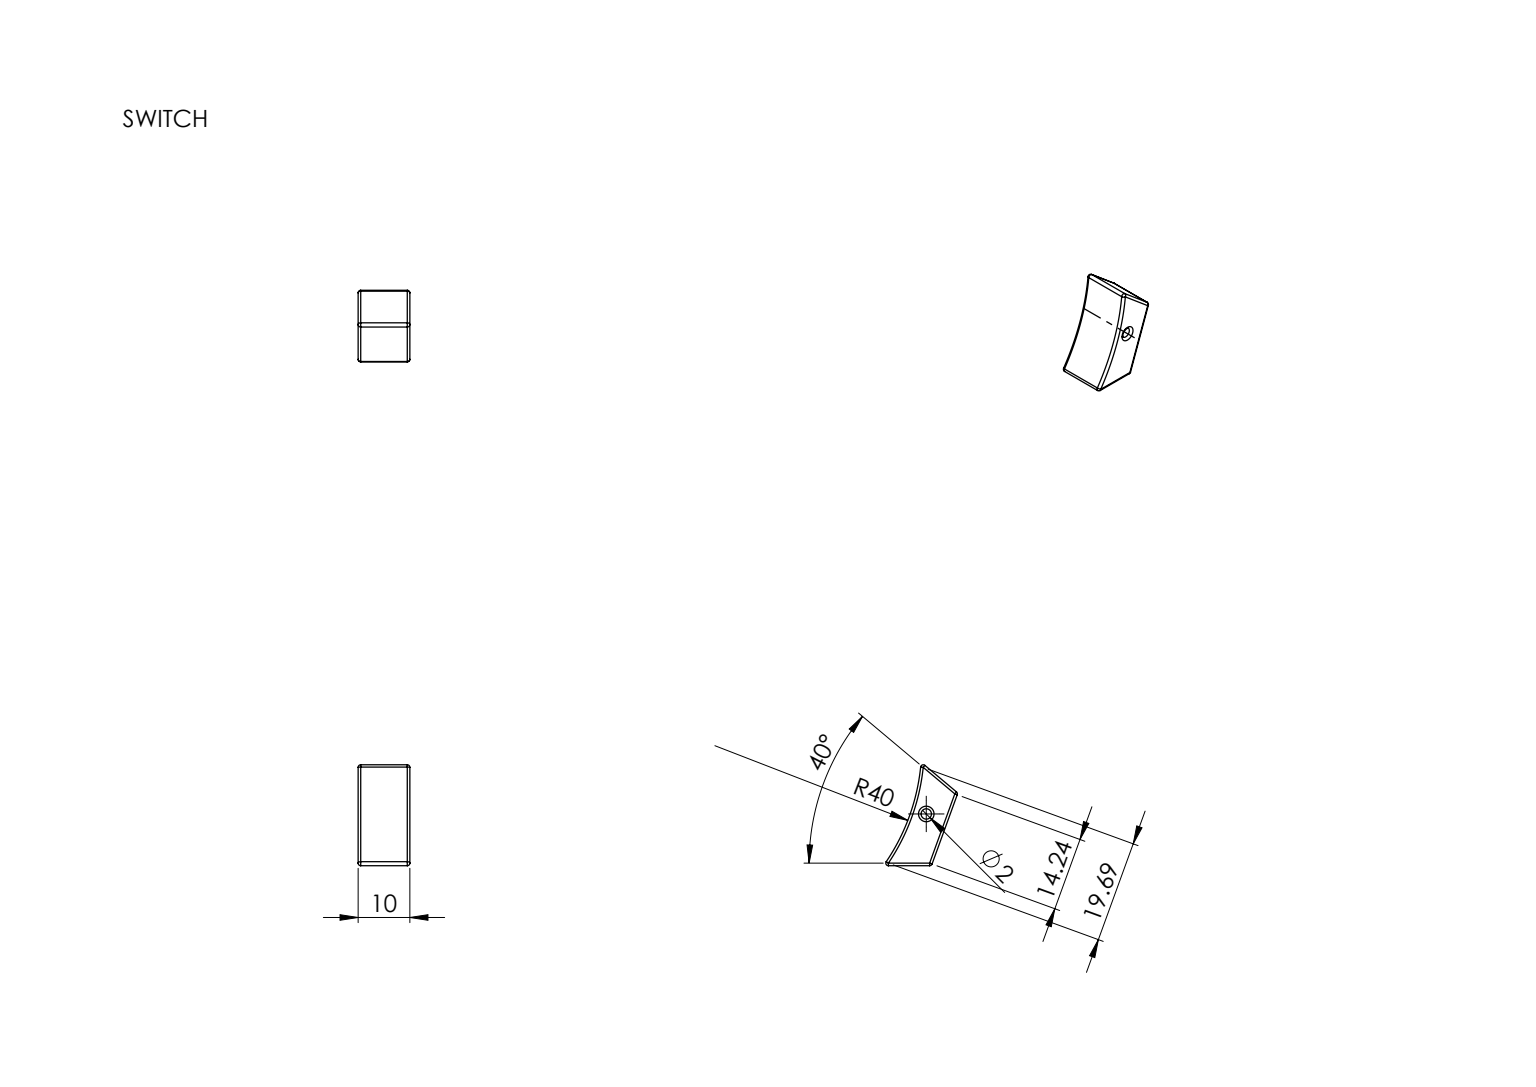
ISO-10303-21;
HEADER;
FILE_DESCRIPTION (('STEP AP214'),
    '1' );
FILE_NAME ('Switch.step',
    '2026-10-04T13:31:42',
    ( '' ),
    ( '' ),
    'SwSTEP 2.0',
    'SolidWorks 2026',
    '' );
FILE_SCHEMA (( 'AUTOMOTIVE_DESIGN' ));
ENDSEC;

DATA;
#378=FACE_OUTER_BOUND ( 'NONE', #8839, .T. ) ;
#599=EDGE_CURVE ( 'NONE', #42462, #65926, #197470, .T. ) ;
#924=FACE_BOUND ( 'NONE', #178509, .T. ) ;
#1415=VERTEX_POINT ( 'NONE', #56964 ) ;
#1694=DIRECTION ( 'NONE',  ( 1.000000000000000000, 0.000000000000000000, -0.000000000000000000 ) ) ;
#1868=FACE_OUTER_BOUND ( 'NONE', #166626, .T. ) ;
#1972=CARTESIAN_POINT ( 'NONE',  ( 4.500000000000000888, -126.2936762853306902, 8.011306146643438097 ) ) ;
#2002=TOROIDAL_SURFACE ( 'NONE', #8512, 40.49999999999999289, 0.5000000000000000000 ) ;
#2126=FACE_OUTER_BOUND ( 'NONE', #140551, .T. ) ;
#2579=SURFACE_SIDE_STYLE ('',( #75448 ) ) ;
#2662=EDGE_LOOP ( 'NONE', ( #45263, #157409, #181382, #132862 ) ) ;
#2725=ORIENTED_EDGE ( 'NONE', *, *, #92972, .T. ) ;
#2819=EDGE_CURVE ( 'NONE', #146728, #77030, #14249, .T. ) ;
#2914=EDGE_CURVE ( 'NONE', #152202, #186287, #21179, .T. ) ;
#3036=DIRECTION ( 'NONE',  ( 0.000000000000000000, 0.000000000000000000, 1.000000000000000000 ) ) ;
#3292=EDGE_LOOP ( 'NONE', ( #165342, #121879, #135522, #133598 ) ) ;
#4504=CIRCLE ( 'NONE', #14199, 0.5000000000000005551 ) ;
#4556=DIRECTION ( 'NONE',  ( 0.000000000000000000, 1.000000000000000000, 0.000000000000000000 ) ) ;
#4699=STYLED_ITEM ( 'NONE', ( #184623 ), #5735 ) ;
#4972=VERTEX_POINT ( 'NONE', #44107 ) ;
#4989=CIRCLE ( 'NONE', #117593, 0.5000000000000004441 ) ;
#4990=ORIENTED_EDGE ( 'NONE', *, *, #133302, .T. ) ;
#5167=AXIS2_PLACEMENT_3D ( 'NONE', #72107, #11455, #147960 ) ;
#5192=CYLINDRICAL_SURFACE ( 'NONE', #117906, 0.5000000000000004441 ) ;
#5395=CARTESIAN_POINT ( 'NONE',  ( 4.500000000000000888, -130.0000000000000000, 12.49999999999999645 ) ) ;
#5599=AXIS2_PLACEMENT_3D ( 'NONE', #147019, #83327, #192528 ) ;
#5735=MANIFOLD_SOLID_BREP ( 'Fillet1', #195579 ) ;
#5844=DIRECTION ( 'NONE',  ( 0.000000000000000000, -0.9396926207859095381, 0.3420201433256656043 ) ) ;
#5989=CARTESIAN_POINT ( 'NONE',  ( -4.500000000000001776, -120.9970989573719038, 14.58956564881030182 ) ) ;
#6194=DIRECTION ( 'NONE',  ( 0.000000000000000000, 0.000000000000000000, 1.000000000000000000 ) ) ;
#6269=TOROIDAL_SURFACE ( 'NONE', #22456, 1.500000000000001776, 0.5000000000000000000 ) ;
#6944=CARTESIAN_POINT ( 'NONE',  ( 5.000000000000000000, -139.5000000000000000, 21.32407087589996308 ) ) ;
#7444=UNCERTAINTY_MEASURE_WITH_UNIT (LENGTH_MEASURE( 1.000000000000000082E-05 ), #170444, 'distance_accuracy_value', 'NONE');
#7466=ADVANCED_FACE ( 'NONE', ( #43887 ), #170200, .T. ) ;
#7837=FACE_OUTER_BOUND ( 'NONE', #8950, .T. ) ;
#7865=VECTOR ( 'NONE', #42257, 1000.000000000000114 ) ;
#8043=TOROIDAL_SURFACE ( 'NONE', #111384, 40.49999999999999289, 0.5000000000000000000 ) ;
#8205=FACE_OUTER_BOUND ( 'NONE', #27654, .T. ) ;
#8263=AXIS2_PLACEMENT_3D ( 'NONE', #15571, #11625, #198607 ) ;
#8512=AXIS2_PLACEMENT_3D ( 'NONE', #12362, #182190, #164046 ) ;
#8537=EDGE_CURVE ( 'NONE', #42462, #143427, #37181, .T. ) ;
#8839=EDGE_LOOP ( 'NONE', ( #48329, #140518, #172705 ) ) ;
#8918=LINE ( 'NONE', #11931, #7865 ) ;
#8950=EDGE_LOOP ( 'NONE', ( #154421, #38535, #18480, #137340 ) ) ;
#8972=CARTESIAN_POINT ( 'NONE',  ( 5.000000000000000888, -130.0000000000000000, 15.50000000000000000 ) ) ;
#9109=CIRCLE ( 'NONE', #176970, 0.4999999999999945044 ) ;
#9224=DIRECTION ( 'NONE',  ( 0.000000000000000000, 0.000000000000000000, 1.000000000000000000 ) ) ;
#9776=AXIS2_PLACEMENT_3D ( 'NONE', #62764, #199314, #60780 ) ;
#10252=FACE_OUTER_BOUND ( 'NONE', #20116, .T. ) ;
#10443=DIRECTION ( 'NONE',  ( -1.000000000000000000, 0.000000000000000000, 0.000000000000000000 ) ) ;
#10604=EDGE_CURVE ( 'NONE', #65926, #12274, #14541, .T. ) ;
#10968=AXIS2_PLACEMENT_3D ( 'NONE', #157679, #65654, #190998 ) ;
#11186=EDGE_LOOP ( 'NONE', ( #162167, #2725, #62094, #31894 ) ) ;
#11257=DIRECTION ( 'NONE',  ( -1.000000000000000000, -0.000000000000000000, -0.000000000000000000 ) ) ;
#11430=AXIS2_PLACEMENT_3D ( 'NONE', #150249, #119893, #136057 ) ;
#11455=DIRECTION ( 'NONE',  ( -1.000000000000000000, 0.000000000000000000, 0.000000000000000000 ) ) ;
#11482=ADVANCED_FACE ( 'NONE', ( #124482, #93138 ), #137663, .T. ) ;
#11510=ORIENTED_EDGE ( 'NONE', *, *, #66871, .F. ) ;
#11512=ORIENTED_EDGE ( 'NONE', *, *, #90150, .F. ) ;
#11532=VECTOR ( 'NONE', #105037, 1000.000000000000000 ) ;
#11625=DIRECTION ( 'NONE',  ( 0.000000000000000000, 1.000000000000000000, 0.000000000000000000 ) ) ;
#11931=CARTESIAN_POINT ( 'NONE',  ( 4.500000000000000888, -120.0000000000000142, 14.99999999999998757 ) ) ;
#11948=CARTESIAN_POINT ( 'NONE',  ( -4.500000000000001776, -120.0000000000000142, 14.99999999999998757 ) ) ;
#12274=VERTEX_POINT ( 'NONE', #56627 ) ;
#12362=CARTESIAN_POINT ( 'NONE',  ( 4.500000000000000888, -116.8122400552013431, 54.87277500418469600 ) ) ;
#12697=CARTESIAN_POINT ( 'NONE',  ( -4.500000000000001776, -130.0000000000000000, 13.99999999999999822 ) ) ;
#12975=DIRECTION ( 'NONE',  ( -0.000000000000000000, -0.000000000000000000, 1.000000000000000000 ) ) ;
#13394=EDGE_LOOP ( 'NONE', ( #49175, #4990, #164479 ) ) ;
#13564=CARTESIAN_POINT ( 'NONE',  ( 4.500000000000000888, -140.0000000000000000, 13.35010376910484275 ) ) ;
#13630=ORIENTED_EDGE ( 'NONE', *, *, #118352, .T. ) ;
#13918=ORIENTED_EDGE ( 'NONE', *, *, #21608, .F. ) ;
#13975=CARTESIAN_POINT ( 'NONE',  ( -4.500000000000001776, -130.0000000000000000, 12.49999999999999645 ) ) ;
#14194=ORIENTED_EDGE ( 'NONE', *, *, #117570, .F. ) ;
#14199=AXIS2_PLACEMENT_3D ( 'NONE', #66248, #145074, #177443 ) ;
#14220=( LENGTH_UNIT ( ) NAMED_UNIT ( * ) SI_UNIT ( .MILLI., .METRE. ) );
#14249=CIRCLE ( 'NONE', #127243, 1.500000000000001332 ) ;
#14258=MECHANICAL_DESIGN_GEOMETRIC_PRESENTATION_REPRESENTATION('',(#166125),#191927);
#14420=CARTESIAN_POINT ( 'NONE',  ( -5.000000000000000000, -139.8289899283371653, 13.46984631039294200 ) ) ;
#14468=ORIENTED_EDGE ( 'NONE', *, *, #106967, .T. ) ;
#14541=CIRCLE ( 'NONE', #66196, 0.5000000000000004441 ) ;
#14977=DIRECTION ( 'NONE',  ( 0.000000000000000000, 1.000000000000000000, 1.224646799147353207E-16 ) ) ;
#15128=DIRECTION ( 'NONE',  ( -3.469446951953611033E-15, 0.000000000000000000, 1.000000000000000000 ) ) ;
#15407=SPHERICAL_SURFACE ( 'NONE', #19151, 0.5000000000000000000 ) ;
#15492=DIRECTION ( 'NONE',  ( 0.000000000000000000, 0.6427876096865403621, 0.7660444431189770143 ) ) ;
#15549=DIRECTION ( 'NONE',  ( -6.938893903907222067E-15, 0.000000000000000000, 1.000000000000000000 ) ) ;
#15571=CARTESIAN_POINT ( 'NONE',  ( -4.500000000000000888, -139.5000000000000000, 21.32407087589996308 ) ) ;
#15773=FILL_AREA_STYLE_COLOUR ( '', #114395 ) ;
#16484=ORIENTED_EDGE ( 'NONE', *, *, #8537, .T. ) ;
#16488=ORIENTED_EDGE ( 'NONE', *, *, #50912, .T. ) ;
#16517=DIRECTION ( 'NONE',  ( -1.000000000000000000, -0.000000000000000000, -0.000000000000000000 ) ) ;
#16873=CARTESIAN_POINT ( 'NONE',  ( -4.500000000000000888, -139.5000000000000000, 13.35010376910484275 ) ) ;
#17153=PLANE ( 'NONE',  #118219 ) ;
#17200=DIRECTION ( 'NONE',  ( 1.387778780781443782E-14, -0.7660444431189784575, 0.6427876096865388078 ) ) ;
#17217=DIRECTION ( 'NONE',  ( 1.000000000000000000, 0.000000000000000000, -0.000000000000000000 ) ) ;
#17276=CARTESIAN_POINT ( 'NONE',  ( 5.000000000000000000, -130.0000000000000000, 13.99999999999999822 ) ) ;
#17558=DIRECTION ( 'NONE',  ( 1.000000000000000000, 0.000000000000000000, -0.000000000000000000 ) ) ;
#17604=VERTEX_POINT ( 'NONE', #91227 ) ;
#17861=ADVANCED_FACE ( 'NONE', ( #8205 ), #5192, .T. ) ;
#17963=ADVANCED_FACE ( 'NONE', ( #35547 ), #8043, .T. ) ;
#18372=ORIENTED_EDGE ( 'NONE', *, *, #106434, .T. ) ;
#18480=ORIENTED_EDGE ( 'NONE', *, *, #90150, .T. ) ;
#18488=EDGE_CURVE ( 'NONE', #185765, #87616, #87045, .T. ) ;
#18872=DIRECTION ( 'NONE',  ( 0.000000000000000000, 0.000000000000000000, 1.000000000000000000 ) ) ;
#19050=DIRECTION ( 'NONE',  ( -1.000000000000000000, -0.000000000000000000, -0.000000000000000000 ) ) ;
#19151=AXIS2_PLACEMENT_3D ( 'NONE', #140725, #139720, #123555 ) ;
#19213=ORIENTED_EDGE ( 'NONE', *, *, #185215, .T. ) ;
#19550=PRODUCT_DEFINITION_SHAPE ( 'NONE', 'NONE',  #75840 ) ;
#20004=ORIENTED_EDGE ( 'NONE', *, *, #22636, .F. ) ;
#20065=PRODUCT_DEFINITION_CONTEXT ( 'detailed design', #129482, 'design' ) ;
#20116=EDGE_LOOP ( 'NONE', ( #193049, #66892, #148714, #150773 ) ) ;
#20571=DIRECTION ( 'NONE',  ( 0.000000000000000000, 1.000000000000000000, 1.224646799147353207E-16 ) ) ;
#20610=EDGE_CURVE ( 'NONE', #35288, #152202, #4989, .T. ) ;
#20936=FACE_OUTER_BOUND ( 'NONE', #21633, .T. ) ;
#21179=CIRCLE ( 'NONE', #85400, 1.000000000000000888 ) ;
#21487=DIRECTION ( 'NONE',  ( 0.000000000000000000, 0.000000000000000000, 1.000000000000000000 ) ) ;
#21528=DIRECTION ( 'NONE',  ( 0.000000000000000000, 0.000000000000000000, 1.000000000000000000 ) ) ;
#21608=EDGE_CURVE ( 'NONE', #17604, #49235, #69530, .T. ) ;
#21633=EDGE_LOOP ( 'NONE', ( #84606, #123613, #121849, #136515 ) ) ;
#21641=AXIS2_PLACEMENT_3D ( 'NONE', #143178, #142191, #188721 ) ;
#21673=CARTESIAN_POINT ( 'NONE',  ( -4.500000000000001776, -140.0000000000000000, 12.99999999999998224 ) ) ;
#22375=CARTESIAN_POINT ( 'NONE',  ( 4.500000000000000888, -139.2199041982123617, 21.73825240834792893 ) ) ;
#22456=AXIS2_PLACEMENT_3D ( 'NONE', #131667, #193349, #21487 ) ;
#22636=EDGE_CURVE ( 'NONE', #198944, #186287, #155898, .T. ) ;
#23392=DIRECTION ( 'NONE',  ( -6.938893903907234689E-15, -0.000000000000000000, -1.000000000000000000 ) ) ;
#23582=ORIENTED_EDGE ( 'NONE', *, *, #188483, .T. ) ;
#23746=CIRCLE ( 'NONE', #39898, 0.5000000000000004441 ) ;
#24011=DIRECTION ( 'NONE',  ( -5.690990215841557531E-14, -0.9396926207859042091, 0.3420201433256805368 ) ) ;
#24115=AXIS2_PLACEMENT_3D ( 'NONE', #59003, #135864, #120669 ) ;
#24413=ORIENTED_EDGE ( 'NONE', *, *, #109644, .T. ) ;
#24683=EDGE_LOOP ( 'NONE', ( #195751, #105223, #94010 ) ) ;
#24698=AXIS2_PLACEMENT_3D ( 'NONE', #120499, #73035, #193375 ) ;
#24883=EDGE_LOOP ( 'NONE', ( #143497, #39612 ) ) ;
#24889=AXIS2_PLACEMENT_3D ( 'NONE', #89830, #120161, #154234 ) ;
#25011=AXIS2_PLACEMENT_3D ( 'NONE', #126547, #96210, #189245 ) ;
#25528=AXIS2_PLACEMENT_3D ( 'NONE', #137746, #95218, #199430 ) ;
#25624=FACE_OUTER_BOUND ( 'NONE', #84344, .T. ) ;
#26835=EDGE_LOOP ( 'NONE', ( #16484, #11512, #112832, #116767 ) ) ;
#26940=CARTESIAN_POINT ( 'NONE',  ( 5.000000000000000000, -139.6710100716628631, 12.88025745871188477 ) ) ;
#27629=DIRECTION ( 'NONE',  ( 0.000000000000000000, -0.5601916035752871892, -0.8283630648959117160 ) ) ;
#27654=EDGE_LOOP ( 'NONE', ( #126119, #152794, #178102, #51671 ) ) ;
#27740=AXIS2_PLACEMENT_3D ( 'NONE', #191960, #177810, #114103 ) ;
#27835=ORIENTED_EDGE ( 'NONE', *, *, #22636, .T. ) ;
#27885=ORIENTED_EDGE ( 'NONE', *, *, #73810, .F. ) ;
#28132=CARTESIAN_POINT ( 'NONE',  ( 5.000000000000000000, -130.0000000000000000, 15.00000000000000000 ) ) ;
#28496=ORIENTED_EDGE ( 'NONE', *, *, #167527, .T. ) ;
#29129=DIRECTION ( 'NONE',  ( 0.000000000000000000, 0.7660444431189601389, -0.6427876096865606792 ) ) ;
#29163=EDGE_LOOP ( 'NONE', ( #53823, #165475, #199587 ) ) ;
#30141=DIRECTION ( 'NONE',  ( 1.000000000000000000, 0.000000000000000000, 0.000000000000000000 ) ) ;
#30227=DIRECTION ( 'NONE',  ( 0.000000000000000000, -0.9396926207859095381, 0.3420201433256656043 ) ) ;
#30328=ORIENTED_EDGE ( 'NONE', *, *, #100701, .F. ) ;
#30750=FACE_OUTER_BOUND ( 'NONE', #102793, .T. ) ;
#31122=DIRECTION ( 'NONE',  ( -0.000000000000000000, -0.6427876096865403621, -0.7660444431189770143 ) ) ;
#31285=PLANE ( 'NONE',  #48341 ) ;
#31292=CARTESIAN_POINT ( 'NONE',  ( -4.500000000000000888, -126.1226662136678272, 8.481152457036388981 ) ) ;
#31777=ORIENTED_EDGE ( 'NONE', *, *, #169612, .T. ) ;
#31894=ORIENTED_EDGE ( 'NONE', *, *, #189089, .F. ) ;
#32046=FACE_OUTER_BOUND ( 'NONE', #54152, .T. ) ;
#32685=CARTESIAN_POINT ( 'NONE',  ( -4.500000000000000888, -120.9970989573719038, 14.58956564881029827 ) ) ;
#33820=ORIENTED_EDGE ( 'NONE', *, *, #148013, .T. ) ;
#33975=ADVANCED_FACE ( 'NONE', ( #68246 ), #36908, .T. ) ;
#34211=DIRECTION ( 'NONE',  ( -1.000000000000000000, -0.000000000000000000, 0.000000000000000000 ) ) ;
#34369=( LENGTH_UNIT ( ) NAMED_UNIT ( * ) SI_UNIT ( .MILLI., .METRE. ) );
#34377=VERTEX_POINT ( 'NONE', #46883 ) ;
#34659=AXIS2_PLACEMENT_3D ( 'NONE', #187400, #61040, #153051 ) ;
#34819=CARTESIAN_POINT ( 'NONE',  ( -4.500000000000001776, -130.0000000000000000, 15.50000000000000000 ) ) ;
#35196=DIRECTION ( 'NONE',  ( 0.000000000000000000, -0.3420201433256804813, -0.9396926207859040980 ) ) ;
#35288=VERTEX_POINT ( 'NONE', #83166 ) ;
#35509=ORIENTED_EDGE ( 'NONE', *, *, #47680, .F. ) ;
#35547=FACE_OUTER_BOUND ( 'NONE', #64964, .T. ) ;
#35564=ORIENTED_EDGE ( 'NONE', *, *, #133302, .F. ) ;
#35577=ORIENTED_EDGE ( 'NONE', *, *, #98904, .F. ) ;
#36610=CIRCLE ( 'NONE', #110819, 0.5000000000000004441 ) ;
#36908=SPHERICAL_SURFACE ( 'NONE', #172699, 0.5000000000000000000 ) ;
#37181=CIRCLE ( 'NONE', #88878, 0.5000000000000004441 ) ;
#37464=VERTEX_POINT ( 'NONE', #52389 ) ;
#37485=CARTESIAN_POINT ( 'NONE',  ( 5.000000000000000000, -140.0000000000000000, 13.35010376910484275 ) ) ;
#37642=TOROIDAL_SURFACE ( 'NONE', #24698, 1.500000000000001776, 0.5000000000000000000 ) ;
#38193=PLANE ( 'NONE',  #69125 ) ;
#38371=CARTESIAN_POINT ( 'NONE',  ( -5.000000000000000000, -139.5000000000000000, 13.35010376910484631 ) ) ;
#38535=ORIENTED_EDGE ( 'NONE', *, *, #142437, .T. ) ;
#38582=DIRECTION ( 'NONE',  ( 0.000000000000000000, 0.000000000000000000, 1.000000000000000000 ) ) ;
#39277=VERTEX_POINT ( 'NONE', #184133 ) ;
#39612=ORIENTED_EDGE ( 'NONE', *, *, #129926, .T. ) ;
#39762=ORIENTED_EDGE ( 'NONE', *, *, #185215, .F. ) ;
#39811=CARTESIAN_POINT ( 'NONE',  ( 5.000000000000000000, -116.8122400552013431, 54.87277500418469600 ) ) ;
#39898=AXIS2_PLACEMENT_3D ( 'NONE', #85387, #97542, #114733 ) ;
#40036=AXIS2_PLACEMENT_3D ( 'NONE', #113385, #86057, #98197 ) ;
#40095=CARTESIAN_POINT ( 'NONE',  ( 4.500000000000000888, -126.1226662136678556, 8.481152457036394310 ) ) ;
#40269=AXIS2_PLACEMENT_3D ( 'NONE', #40095, #67436, #129093 ) ;
#40522=CIRCLE ( 'NONE', #153513, 0.5000000000000004441 ) ;
#40998=AXIS2_PLACEMENT_3D ( 'NONE', #133958, #54112, #118796 ) ;
#41140=VECTOR ( 'NONE', #193532, 1000.000000000000000 ) ;
#41555=CARTESIAN_POINT ( 'NONE',  ( 5.000000000000000000, -140.0000000000000000, 21.32407087589996308 ) ) ;
#42011=ORIENTED_EDGE ( 'NONE', *, *, #151687, .T. ) ;
#42047=EDGE_LOOP ( 'NONE', ( #13918, #194517, #91810, #48248 ) ) ;
#42257=DIRECTION ( 'NONE',  ( -0.000000000000000000, -0.6427876096865403621, -0.7660444431189770143 ) ) ;
#42379=DIRECTION ( 'NONE',  ( 0.000000000000000000, -3.469446951953611428E-15, -1.000000000000000000 ) ) ;
#42462=VERTEX_POINT ( 'NONE', #111627 ) ;
#42923=DIRECTION ( 'NONE',  ( 0.000000000000000000, 0.9396926207859095381, -0.3420201433256656043 ) ) ;
#42957=VECTOR ( 'NONE', #136873, 1000.000000000000000 ) ;
#43297=DIRECTION ( 'NONE',  ( 0.000000000000000000, 0.000000000000000000, -1.000000000000000000 ) ) ;
#43658=CARTESIAN_POINT ( 'NONE',  ( 5.000000000000000000, -126.2936762853306902, 8.011306146643438097 ) ) ;
#43887=FACE_OUTER_BOUND ( 'NONE', #24683, .T. ) ;
#44019=DIRECTION ( 'NONE',  ( 0.000000000000000000, 0.000000000000000000, 1.000000000000000000 ) ) ;
#44107=CARTESIAN_POINT ( 'NONE',  ( -4.500000000000001776, -140.0000000000000000, 13.35010376910484275 ) ) ;
#44161=ADVANCED_FACE ( 'NONE', ( #7837 ), #38193, .F. ) ;
#44289=DIRECTION ( 'NONE',  ( 1.075492293517917348E-15, -0.9946471445771457587, 0.1033298494363120851 ) ) ;
#44589=CIRCLE ( 'NONE', #105920, 0.5000000000000004441 ) ;
#44837=LINE ( 'NONE', #168170, #143440 ) ;
#45263=ORIENTED_EDGE ( 'NONE', *, *, #151687, .F. ) ;
#45318=CYLINDRICAL_SURFACE ( 'NONE', #112421, 0.4999999999999995559 ) ;
#45746=CARTESIAN_POINT ( 'NONE',  ( -4.500000000000001776, -139.5000000000000000, 21.32407087589996664 ) ) ;
#46137=ORIENTED_EDGE ( 'NONE', *, *, #21608, .T. ) ;
#46278=LINE ( 'NONE', #199970, #98639 ) ;
#46448=DIRECTION ( 'NONE',  ( -1.000000000000000000, -0.000000000000000000, 0.000000000000000000 ) ) ;
#46562=EDGE_LOOP ( 'NONE', ( #140120, #80075, #117583, #109420 ) ) ;
#46883=CARTESIAN_POINT ( 'NONE',  ( 5.000000000000000000, -139.5000000000000000, 13.35010376910484098 ) ) ;
#47107=( NAMED_UNIT ( * ) SI_UNIT ( $, .STERADIAN. ) SOLID_ANGLE_UNIT ( ) );
#47118=EDGE_CURVE ( 'NONE', #49927, #87243, #127276, .T. ) ;
#47498=AXIS2_PLACEMENT_3D ( 'NONE', #165368, #168329, #59154 ) ;
#47680=EDGE_CURVE ( 'NONE', #35288, #198944, #153126, .T. ) ;
#48214=CYLINDRICAL_SURFACE ( 'NONE', #124993, 1.000000000000000888 ) ;
#48248=ORIENTED_EDGE ( 'NONE', *, *, #74471, .F. ) ;
#48329=ORIENTED_EDGE ( 'NONE', *, *, #181003, .F. ) ;
#48341=AXIS2_PLACEMENT_3D ( 'NONE', #79770, #46448, #141440 ) ;
#48553=( NAMED_UNIT ( * ) SI_UNIT ( $, .STERADIAN. ) SOLID_ANGLE_UNIT ( ) );
#48868=CARTESIAN_POINT ( 'NONE',  ( -4.500000000000000888, -139.5000000000000000, 21.32407087589996308 ) ) ;
#49175=ORIENTED_EDGE ( 'NONE', *, *, #193069, .T. ) ;
#49235=VERTEX_POINT ( 'NONE', #56515 ) ;
#49270=CARTESIAN_POINT ( 'NONE',  ( -5.000000000000000000, -126.3477085785529823, 8.212957410198603370 ) ) ;
#49850=LINE ( 'NONE', #52822, #54817 ) ;
#49927=VERTEX_POINT ( 'NONE', #94796 ) ;
#50180=AXIS2_PLACEMENT_3D ( 'NONE', #69708, #42379, #101030 ) ;
#50205=DIRECTION ( 'NONE',  ( 0.000000000000000000, 0.000000000000000000, 1.000000000000000000 ) ) ;
#50472=ORIENTED_EDGE ( 'NONE', *, *, #174667, .F. ) ;
#50504=AXIS2_PLACEMENT_3D ( 'NONE', #179746, #130190, #191886 ) ;
#50527=DIRECTION ( 'NONE',  ( 2.126200446592120372E-14, -0.6427876096865389188, -0.7660444431189784575 ) ) ;
#50546=EDGE_CURVE ( 'NONE', #72196, #146762, #166148, .T. ) ;
#50743=EDGE_CURVE ( 'NONE', #37464, #49927, #44837, .T. ) ;
#50912=EDGE_CURVE ( 'NONE', #39277, #90572, #153271, .T. ) ;
#51035=CARTESIAN_POINT ( 'NONE',  ( 5.000000000000000000, -139.5000000000000000, 21.32407087589995953 ) ) ;
#51095=CARTESIAN_POINT ( 'NONE',  ( 4.500000000000000888, -139.5000000000000000, 21.32407087589996308 ) ) ;
#51671=ORIENTED_EDGE ( 'NONE', *, *, #74956, .F. ) ;
#51718=DIRECTION ( 'NONE',  ( 1.000000000000000000, 0.000000000000000000, -6.938893903907222067E-15 ) ) ;
#52273=SHAPE_DEFINITION_REPRESENTATION ( #19550, #125845 ) ;
#52389=CARTESIAN_POINT ( 'NONE',  ( 5.000000000000000000, -126.1226662136678272, 8.481152457036383652 ) ) ;
#52459=CYLINDRICAL_SURFACE ( 'NONE', #70160, 0.5000000000000004441 ) ;
#52697=AXIS2_PLACEMENT_3D ( 'NONE', #13975, #14977, #168645 ) ;
#52822=CARTESIAN_POINT ( 'NONE',  ( 5.000000000000000000, -139.5000000000000000, 21.82407087589996308 ) ) ;
#53066=DIRECTION ( 'NONE',  ( -3.469446951953611033E-15, 0.000000000000000000, -1.000000000000000000 ) ) ;
#53098=DIRECTION ( 'NONE',  ( 0.000000000000000000, 0.3420201433257384349, 0.9396926207858830038 ) ) ;
#53331=CARTESIAN_POINT ( 'NONE',  ( -4.500000000000001776, -126.1226662136678556, 8.481152457036394310 ) ) ;
#53338=VECTOR ( 'NONE', #109893, 1000.000000000000000 ) ;
#53823=ORIENTED_EDGE ( 'NONE', *, *, #77310, .T. ) ;
#53964=ADVANCED_FACE ( 'NONE', ( #156147 ), #129763, .T. ) ;
#54112=DIRECTION ( 'NONE',  ( 0.000000000000000000, -0.8283630648959183773, 0.5601916035752775302 ) ) ;
#54152=EDGE_LOOP ( 'NONE', ( #20004, #35509, #94186, #134138 ) ) ;
#54419=CARTESIAN_POINT ( 'NONE',  ( 4.500000000000000888, -140.0000000000000000, 12.99999999999998224 ) ) ;
#54817=VECTOR ( 'NONE', #141847, 1000.000000000000000 ) ;
#54933=AXIS2_PLACEMENT_3D ( 'NONE', #17276, #94099, #198316 ) ;
#56261=VECTOR ( 'NONE', #149965, 1000.000000000000000 ) ;
#56515=CARTESIAN_POINT ( 'NONE',  ( 4.500000000000000888, -130.0000000000000000, 15.00000000000000000 ) ) ;
#56627=CARTESIAN_POINT ( 'NONE',  ( -4.500000000000001776, -139.6710100716628631, 12.88025745871188654 ) ) ;
#56756=DIRECTION ( 'NONE',  ( -3.469446951953611033E-15, 0.000000000000000000, -1.000000000000000000 ) ) ;
#56771=EDGE_LOOP ( 'NONE', ( #163725, #183501, #98509 ) ) ;
#56964=CARTESIAN_POINT ( 'NONE',  ( -4.500000000000001776, -125.7396439921083555, 8.159758652193113804 ) ) ;
#57428=CARTESIAN_POINT ( 'NONE',  ( -4.500000000000001776, -120.9454340326537505, 15.08688922109887187 ) ) ;
#57457=EDGE_LOOP ( 'NONE', ( #14194, #92671, #33820 ) ) ;
#58648=DIRECTION ( 'NONE',  ( 0.000000000000000000, 1.000000000000000000, 0.000000000000000000 ) ) ;
#58736=EDGE_CURVE ( 'NONE', #124967, #80629, #98541, .T. ) ;
#59003=CARTESIAN_POINT ( 'NONE',  ( 4.500000000000000888, -139.5000000000000000, 13.35010376910484275 ) ) ;
#59154=DIRECTION ( 'NONE',  ( 0.000000000000000000, 0.000000000000000000, 1.000000000000000000 ) ) ;
#59375=AXIS2_PLACEMENT_3D ( 'NONE', #111759, #4556, #53066 ) ;
#59827=DIRECTION ( 'NONE',  ( 0.000000000000000000, 0.000000000000000000, 1.000000000000000000 ) ) ;
#60083=SPHERICAL_SURFACE ( 'NONE', #91461, 0.5000000000000000000 ) ;
#60362=VECTOR ( 'NONE', #72715, 1000.000000000000000 ) ;
#60549=CYLINDRICAL_SURFACE ( 'NONE', #112279, 0.5000000000000037748 ) ;
#60666=CARTESIAN_POINT ( 'NONE',  ( 5.000000000000000000, -120.9454340326537505, 15.08688922109886832 ) ) ;
#60732=AXIS2_PLACEMENT_3D ( 'NONE', #31292, #58648, #15128 ) ;
#60780=DIRECTION ( 'NONE',  ( 0.000000000000000000, 0.000000000000000000, -1.000000000000000000 ) ) ;
#61040=DIRECTION ( 'NONE',  ( -1.000000000000000000, -0.000000000000000000, 0.000000000000000000 ) ) ;
#61266=SURFACE_STYLE_USAGE ( .BOTH. , #2579 ) ;
#61485=ADVANCED_FACE ( 'NONE', ( #10252 ), #177111, .F. ) ;
#61711=ADVANCED_FACE ( 'NONE', ( #103253 ), #130569, .T. ) ;
#62050=DIRECTION ( 'NONE',  ( 7.973251674720317682E-15, -0.6427876096865524636, -0.7660444431189670222 ) ) ;
#62094=ORIENTED_EDGE ( 'NONE', *, *, #121277, .T. ) ;
#62487=ORIENTED_EDGE ( 'NONE', *, *, #116810, .T. ) ;
#62627=EDGE_CURVE ( 'NONE', #87358, #84042, #144207, .T. ) ;
#62764=CARTESIAN_POINT ( 'NONE',  ( 4.500000000000000888, -126.1226662136678272, 8.481152457036388981 ) ) ;
#63549=DIRECTION ( 'NONE',  ( 0.000000000000000000, -0.7660444431189771253, 0.6427876096865404731 ) ) ;
#63761=ADVANCED_FACE ( 'NONE', ( #180869 ), #80358, .T. ) ;
#63808=DIRECTION ( 'NONE',  ( 0.000000000000000000, 0.000000000000000000, 1.000000000000000000 ) ) ;
#63974=ORIENTED_EDGE ( 'NONE', *, *, #168190, .F. ) ;
#64031=SPHERICAL_SURFACE ( 'NONE', #131523, 0.5000000000000000000 ) ;
#64259=( NAMED_UNIT ( * ) PLANE_ANGLE_UNIT ( ) SI_UNIT ( $, .RADIAN. ) );
#64964=EDGE_LOOP ( 'NONE', ( #18372, #154496, #27885, #105016 ) ) ;
#65654=DIRECTION ( 'NONE',  ( -1.000000000000000000, 0.000000000000000000, -0.000000000000000000 ) ) ;
#65926=VERTEX_POINT ( 'NONE', #38371 ) ;
#66078=ORIENTED_EDGE ( 'NONE', *, *, #50743, .T. ) ;
#66196=AXIS2_PLACEMENT_3D ( 'NONE', #67026, #142864, #144857 ) ;
#66248=CARTESIAN_POINT ( 'NONE',  ( -4.500000000000000888, -120.9970989573719038, 14.58956564881029472 ) ) ;
#66523=PLANE ( 'NONE',  #99433 ) ;
#66811=TOROIDAL_SURFACE ( 'NONE', #21641, 1.500000000000001776, 0.5000000000000000000 ) ;
#66871=EDGE_CURVE ( 'NONE', #34377, #37464, #87856, .T. ) ;
#66892=ORIENTED_EDGE ( 'NONE', *, *, #74956, .T. ) ;
#66950=VERTEX_POINT ( 'NONE', #76808 ) ;
#67026=CARTESIAN_POINT ( 'NONE',  ( -4.500000000000000888, -139.5000000000000000, 13.35010376910484631 ) ) ;
#67436=DIRECTION ( 'NONE',  ( 1.000000000000000000, 0.000000000000000000, 0.000000000000000000 ) ) ;
#67613=DIRECTION ( 'NONE',  ( 0.000000000000000000, -0.000000000000000000, 1.000000000000000000 ) ) ;
#67627=DIRECTION ( 'NONE',  ( 0.000000000000000000, 0.000000000000000000, 1.000000000000000000 ) ) ;
#68079=ORIENTED_EDGE ( 'NONE', *, *, #142437, .F. ) ;
#68111=DIRECTION ( 'NONE',  ( 0.000000000000000000, 0.7660444431189784575, -0.6427876096865388078 ) ) ;
#68246=FACE_OUTER_BOUND ( 'NONE', #153423, .T. ) ;
#68434=DIRECTION ( 'NONE',  ( 0.000000000000000000, 0.6427876096865404731, 0.7660444431189771253 ) ) ;
#68789=EDGE_CURVE ( 'NONE', #1415, #84042, #150452, .T. ) ;
#68875=CARTESIAN_POINT ( 'NONE',  ( -4.500000000000001776, -116.8122400552013431, 54.87277500418469600 ) ) ;
#69125=AXIS2_PLACEMENT_3D ( 'NONE', #173731, #69523, #5844 ) ;
#69440=DIRECTION ( 'NONE',  ( 0.000000000000000000, -0.7660444431189766812, 0.6427876096865408062 ) ) ;
#69523=DIRECTION ( 'NONE',  ( -0.000000000000000000, 0.3420201433256656043, 0.9396926207859095381 ) ) ;
#69530=CIRCLE ( 'NONE', #108348, 1.000000000000000888 ) ;
#69705=VECTOR ( 'NONE', #137265, 1000.000000000000000 ) ;
#69708=CARTESIAN_POINT ( 'NONE',  ( 4.500000000000000888, -139.5000000000000000, 13.35010376910484098 ) ) ;
#69885=CARTESIAN_POINT ( 'NONE',  ( -4.500000000000001776, -130.0000000000000000, 13.99999999999999822 ) ) ;
#70112=CARTESIAN_POINT ( 'NONE',  ( -4.500000000000001776, -130.0000000000000000, 12.99999999999999822 ) ) ;
#70160=AXIS2_PLACEMENT_3D ( 'NONE', #6944, #82784, #67627 ) ;
#70263=LINE ( 'NONE', #181445, #193831 ) ;
#70645=ORIENTED_EDGE ( 'NONE', *, *, #137830, .T. ) ;
#70778=ADVANCED_FACE ( 'NONE', ( #155047 ), #105691, .T. ) ;
#70935=ORIENTED_EDGE ( 'NONE', *, *, #145468, .T. ) ;
#71001=DIRECTION ( 'NONE',  ( 0.000000000000000000, 0.000000000000000000, 1.000000000000000000 ) ) ;
#71148=ADVANCED_FACE ( 'NONE', ( #170219 ), #64031, .T. ) ;
#71174=ORIENTED_EDGE ( 'NONE', *, *, #113718, .T. ) ;
#71199=ORIENTED_EDGE ( 'NONE', *, *, #186126, .T. ) ;
#71284=DIRECTION ( 'NONE',  ( 0.000000000000000000, -0.6427876096865287048, -0.7660444431189871173 ) ) ;
#71385=ORIENTED_EDGE ( 'NONE', *, *, #193069, .F. ) ;
#71610=VERTEX_POINT ( 'NONE', #155639 ) ;
#72107=CARTESIAN_POINT ( 'NONE',  ( -4.500000000000001776, -139.5000000000000000, 21.32407087589996308 ) ) ;
#72135=ORIENTED_EDGE ( 'NONE', *, *, #113474, .T. ) ;
#72196=VERTEX_POINT ( 'NONE', #114084 ) ;
#72234=CARTESIAN_POINT ( 'NONE',  ( 5.000000000000000000, -120.6140767358124180, 14.26817184396703020 ) ) ;
#72330=AXIS2_PLACEMENT_3D ( 'NONE', #39811, #194512, #114650 ) ;
#72715=DIRECTION ( 'NONE',  ( 0.000000000000000000, 0.9396926207859095381, -0.3420201433256656043 ) ) ;
#73035=DIRECTION ( 'NONE',  ( -1.000000000000000000, -0.000000000000000000, 0.000000000000000000 ) ) ;
#73810=EDGE_CURVE ( 'NONE', #94299, #66950, #118669, .T. ) ;
#73842=DIRECTION ( 'NONE',  ( 0.000000000000000000, 0.000000000000000000, -1.000000000000000000 ) ) ;
#74408=EDGE_LOOP ( 'NONE', ( #114038, #196910, #108990 ) ) ;
#74471=EDGE_CURVE ( 'NONE', #49235, #77030, #92804, .T. ) ;
#74681=ORIENTED_EDGE ( 'NONE', *, *, #182367, .F. ) ;
#74698=CARTESIAN_POINT ( 'NONE',  ( 5.000000000000000000, -132.8113331068338425, 10.91562811307057679 ) ) ;
#74821=SPHERICAL_SURFACE ( 'NONE', #60732, 0.5000000000000000000 ) ;
#74956=EDGE_CURVE ( 'NONE', #80629, #183542, #165889, .T. ) ;
#75448=SURFACE_STYLE_FILL_AREA ( #156264 ) ;
#75463=CIRCLE ( 'NONE', #10968, 0.5000000000000004441 ) ;
#75639=FACE_OUTER_BOUND ( 'NONE', #127342, .T. ) ;
#75840=PRODUCT_DEFINITION ( 'UNKNOWN', '', #179267, #20065 ) ;
#75889=( NAMED_UNIT ( * ) PLANE_ANGLE_UNIT ( ) SI_UNIT ( $, .RADIAN. ) );
#76311=CARTESIAN_POINT ( 'NONE',  ( 4.500000000000000888, -140.0000000000000000, 21.32407087589996308 ) ) ;
#76495=VECTOR ( 'NONE', #133249, 1000.000000000000000 ) ;
#76561=ADVANCED_FACE ( 'NONE', ( #114117 ), #52459, .T. ) ;
#76790=AXIS2_PLACEMENT_3D ( 'NONE', #121112, #44289, #105947 ) ;
#76808=CARTESIAN_POINT ( 'NONE',  ( -5.000000000000000000, -139.5000000000000000, 21.32407087589995953 ) ) ;
#77030=VERTEX_POINT ( 'NONE', #8972 ) ;
#77300=AXIS2_PLACEMENT_3D ( 'NONE', #130653, #102331, #71001 ) ;
#77310=EDGE_CURVE ( 'NONE', #42462, #1415, #9109, .T. ) ;
#78055=EDGE_CURVE ( 'NONE', #49927, #80629, #89793, .T. ) ;
#78165=DIRECTION ( 'NONE',  ( 0.000000000000000000, 0.000000000000000000, 1.000000000000000000 ) ) ;
#78218=DIRECTION ( 'NONE',  ( 0.000000000000000000, 1.000000000000000000, 0.000000000000000000 ) ) ;
#78635=ORIENTED_EDGE ( 'NONE', *, *, #77310, .F. ) ;
#79224=DIRECTION ( 'NONE',  ( -3.469446951953611033E-15, 0.000000000000000000, -1.000000000000000000 ) ) ;
#79289=ADVANCED_FACE ( 'NONE', ( #199081 ), #60549, .T. ) ;
#79380=ADVANCED_FACE ( 'NONE', ( #1868 ), #66523, .F. ) ;
#79770=CARTESIAN_POINT ( 'NONE',  ( 5.000000000000000000, -116.8122400552013431, 54.87277500418469600 ) ) ;
#79813=ADVANCED_FACE ( 'NONE', ( #126210 ), #156556, .T. ) ;
#80075=ORIENTED_EDGE ( 'NONE', *, *, #95661, .T. ) ;
#80358=CYLINDRICAL_SURFACE ( 'NONE', #24889, 0.5000000000000004441 ) ;
#80629=VERTEX_POINT ( 'NONE', #117016 ) ;
#81459=EDGE_LOOP ( 'NONE', ( #106495, #27835, #99592, #161714 ) ) ;
#82054=AXIS2_PLACEMENT_3D ( 'NONE', #82060, #99242, #83075 ) ;
#82060=CARTESIAN_POINT ( 'NONE',  ( 0.000000000000000000, 0.000000000000000000, 0.000000000000000000 ) ) ;
#82784=DIRECTION ( 'NONE',  ( -1.000000000000000000, -0.000000000000000000, -0.000000000000000000 ) ) ;
#83034=DIRECTION ( 'NONE',  ( -1.000000000000000000, -0.000000000000000000, -0.000000000000000000 ) ) ;
#83075=DIRECTION ( 'NONE',  ( 1.000000000000000000, 0.000000000000000000, 0.000000000000000000 ) ) ;
#83121=VECTOR ( 'NONE', #134560, 1000.000000000000000 ) ;
#83166=CARTESIAN_POINT ( 'NONE',  ( -5.000000000000000888, -130.0000000000000000, 15.50000000000000000 ) ) ;
#83327=DIRECTION ( 'NONE',  ( -1.000000000000000000, -0.000000000000000000, -0.000000000000000000 ) ) ;
#83522=DIRECTION ( 'NONE',  ( 0.000000000000000000, 0.000000000000000000, -1.000000000000000000 ) ) ;
#84042=VERTEX_POINT ( 'NONE', #171637 ) ;
#84282=ADVANCED_FACE ( 'NONE', ( #75639 ), #45318, .T. ) ;
#84344=EDGE_LOOP ( 'NONE', ( #160083, #87947, #35564, #146092 ) ) ;
#84606=ORIENTED_EDGE ( 'NONE', *, *, #168074, .T. ) ;
#85260=LINE ( 'NONE', #115618, #195745 ) ;
#85327=LINE ( 'NONE', #21673, #41140 ) ;
#85387=CARTESIAN_POINT ( 'NONE',  ( 4.500000000000000888, -126.1226662136678556, 8.481152457036394310 ) ) ;
#85400=AXIS2_PLACEMENT_3D ( 'NONE', #69885, #145715, #113377 ) ;
#86057=DIRECTION ( 'NONE',  ( -0.000000000000000000, -6.938893903907222856E-15, -1.000000000000000000 ) ) ;
#86149=CIRCLE ( 'NONE', #40998, 0.5000000000000041078 ) ;
#87045=LINE ( 'NONE', #41555, #159879 ) ;
#87243=VERTEX_POINT ( 'NONE', #51035 ) ;
#87269=DIRECTION ( 'NONE',  ( 0.000000000000000000, 0.000000000000000000, -1.000000000000000000 ) ) ;
#87290=ORIENTED_EDGE ( 'NONE', *, *, #117570, .T. ) ;
#87358=VERTEX_POINT ( 'NONE', #124896 ) ;
#87616=VERTEX_POINT ( 'NONE', #143028 ) ;
#87856=LINE ( 'NONE', #74698, #60362 ) ;
#87947=ORIENTED_EDGE ( 'NONE', *, *, #131422, .F. ) ;
#88430=CARTESIAN_POINT ( 'NONE',  ( 5.000000000000000888, -130.0000000000000000, 12.49999999999999645 ) ) ;
#88735=AXIS2_PLACEMENT_3D ( 'NONE', #32685, #153032, #156016 ) ;
#88765=CARTESIAN_POINT ( 'NONE',  ( -4.500000000000001776, -126.2936762853306902, 8.011306146643438097 ) ) ;
#88851=ORIENTED_EDGE ( 'NONE', *, *, #66871, .T. ) ;
#88878=AXIS2_PLACEMENT_3D ( 'NONE', #53331, #24011, #132178 ) ;
#89075=CARTESIAN_POINT ( 'NONE',  ( -5.000000000000000000, -130.0000000000000000, 13.99999999999999822 ) ) ;
#89793=CIRCLE ( 'NONE', #76790, 0.5000000000000005551 ) ;
#89830=CARTESIAN_POINT ( 'NONE',  ( 5.000000000000000000, -139.5000000000000000, 13.35010376910484275 ) ) ;
#90150=EDGE_CURVE ( 'NONE', #12274, #143427, #70263, .T. ) ;
#90572=VERTEX_POINT ( 'NONE', #13564 ) ;
#91103=DIRECTION ( 'NONE',  ( 0.000000000000000000, 0.000000000000000000, -1.000000000000000000 ) ) ;
#91135=CYLINDRICAL_SURFACE ( 'NONE', #176516, 0.5000000000000004441 ) ;
#91190=ORIENTED_EDGE ( 'NONE', *, *, #188483, .F. ) ;
#91227=CARTESIAN_POINT ( 'NONE',  ( 4.500000000000000888, -130.0000000000000000, 12.99999999999999822 ) ) ;
#91461=AXIS2_PLACEMENT_3D ( 'NONE', #170248, #78218, #79224 ) ;
#91810=ORIENTED_EDGE ( 'NONE', *, *, #116810, .F. ) ;
#92037=SHAPE_REPRESENTATION_RELATIONSHIP ( 'NONE' , 'NONE' ,  #125845, #107481 ) ;
#92344=CIRCLE ( 'NONE', #5167, 0.5000000000000004441 ) ;
#92395=CIRCLE ( 'NONE', #144056, 0.5000000000000004441 ) ;
#92434=EDGE_LOOP ( 'NONE', ( #194625, #117206, #78635, #180537 ) ) ;
#92523=EDGE_CURVE ( 'NONE', #183542, #94299, #158431, .T. ) ;
#92671=ORIENTED_EDGE ( 'NONE', *, *, #50546, .T. ) ;
#92701=CARTESIAN_POINT ( 'NONE',  ( 4.500000000000000888, -130.0000000000000000, 13.99999999999999822 ) ) ;
#92804=CIRCLE ( 'NONE', #25011, 0.5000000000000004441 ) ;
#92972=EDGE_CURVE ( 'NONE', #17604, #186287, #109056, .T. ) ;
#93138=FACE_OUTER_BOUND ( 'NONE', #143331, .T. ) ;
#93336=CYLINDRICAL_SURFACE ( 'NONE', #104284, 1.000000000000000888 ) ;
#93701=FACE_OUTER_BOUND ( 'NONE', #156544, .T. ) ;
#94010=ORIENTED_EDGE ( 'NONE', *, *, #62627, .F. ) ;
#94099=DIRECTION ( 'NONE',  ( -1.000000000000000000, -0.000000000000000000, 0.000000000000000000 ) ) ;
#94186=ORIENTED_EDGE ( 'NONE', *, *, #20610, .T. ) ;
#94218=FACE_OUTER_BOUND ( 'NONE', #74408, .T. ) ;
#94299=VERTEX_POINT ( 'NONE', #173025 ) ;
#94697=CARTESIAN_POINT ( 'NONE',  ( 5.000000000000000000, -130.0000000000000000, 13.99999999999999822 ) ) ;
#94796=CARTESIAN_POINT ( 'NONE',  ( 5.000000000000000000, -120.9970989573719038, 14.58956564881029294 ) ) ;
#95218=DIRECTION ( 'NONE',  ( -1.000000000000000000, 0.000000000000000000, 0.000000000000000000 ) ) ;
#95490=DIRECTION ( 'NONE',  ( 0.000000000000000000, -1.000000000000000000, 0.000000000000000000 ) ) ;
#95661=EDGE_CURVE ( 'NONE', #4972, #90572, #129477, .T. ) ;
#95816=AXIS2_PLACEMENT_3D ( 'NONE', #174230, #17558, #21528 ) ;
#95957=AXIS2_PLACEMENT_3D ( 'NONE', #146270, #68434, #69440 ) ;
#95970=CIRCLE ( 'NONE', #137835, 1.000000000000000888 ) ;
#96210=DIRECTION ( 'NONE',  ( 0.000000000000000000, -1.000000000000000000, 0.000000000000000000 ) ) ;
#97292=ADVANCED_FACE ( 'NONE', ( #924, #157612 ), #31285, .F. ) ;
#97430=CARTESIAN_POINT ( 'NONE',  ( -4.500000000000001776, -120.3830222215595001, 15.32139380484325741 ) ) ;
#97484=FACE_OUTER_BOUND ( 'NONE', #2662, .T. ) ;
#97542=DIRECTION ( 'NONE',  ( 1.000000000000000000, 0.000000000000000000, 0.000000000000000000 ) ) ;
#97927=DIRECTION ( 'NONE',  ( -0.000000000000000000, 1.000000000000000000, 0.000000000000000000 ) ) ;
#98197=DIRECTION ( 'NONE',  ( -1.734723475976805517E-15, -1.000000000000000000, 6.938893903907222067E-15 ) ) ;
#98509=ORIENTED_EDGE ( 'NONE', *, *, #106967, .F. ) ;
#98541=CIRCLE ( 'NONE', #11430, 39.99999999999999289 ) ;
#98571=DIRECTION ( 'NONE',  ( -6.938893903907222067E-15, 0.000000000000000000, -1.000000000000000000 ) ) ;
#98639=VECTOR ( 'NONE', #12975, 1000.000000000000000 ) ;
#98688=CARTESIAN_POINT ( 'NONE',  ( 4.500000000000000888, -139.5000000000000000, 21.32407087589996664 ) ) ;
#98730=AXIS2_PLACEMENT_3D ( 'NONE', #110546, #62050, #141875 ) ;
#98904=EDGE_CURVE ( 'NONE', #143427, #187814, #120481, .T. ) ;
#99118=CIRCLE ( 'NONE', #176665, 0.5000000000000002220 ) ;
#99242=DIRECTION ( 'NONE',  ( 0.000000000000000000, 0.000000000000000000, 1.000000000000000000 ) ) ;
#99433=AXIS2_PLACEMENT_3D ( 'NONE', #188898, #63549, #187906 ) ;
#99592=ORIENTED_EDGE ( 'NONE', *, *, #2914, .F. ) ;
#100238=CARTESIAN_POINT ( 'NONE',  ( 5.000000000000000000, -116.8122400552013431, 54.87277500418469600 ) ) ;
#100701=EDGE_CURVE ( 'NONE', #197216, #71610, #49850, .T. ) ;
#101030=DIRECTION ( 'NONE',  ( 0.000000000000000000, 1.000000000000000000, -3.469446951953611033E-15 ) ) ;
#101230=CARTESIAN_POINT ( 'NONE',  ( 4.500000000000000888, -126.1226662136678272, 8.481152457036388981 ) ) ;
#101443=EDGE_LOOP ( 'NONE', ( #28496, #11510, #71385, #74681 ) ) ;
#101702=CIRCLE ( 'NONE', #182548, 0.5000000000000004441 ) ;
#101748=AXIS2_PLACEMENT_3D ( 'NONE', #97430, #141961, #68111 ) ;
#102331=DIRECTION ( 'NONE',  ( 1.000000000000000000, 0.000000000000000000, -0.000000000000000000 ) ) ;
#102717=ORIENTED_EDGE ( 'NONE', *, *, #47118, .F. ) ;
#102793=EDGE_LOOP ( 'NONE', ( #72135, #87290, #189442 ) ) ;
#103253=FACE_OUTER_BOUND ( 'NONE', #57457, .T. ) ;
#104212=DIRECTION ( 'NONE',  ( -1.000000000000000000, 0.000000000000000000, 0.000000000000000000 ) ) ;
#104284=AXIS2_PLACEMENT_3D ( 'NONE', #153026, #16517, #78165 ) ;
#105016=ORIENTED_EDGE ( 'NONE', *, *, #92523, .F. ) ;
#105037=DIRECTION ( 'NONE',  ( 1.000000000000000000, 0.000000000000000000, 0.000000000000000000 ) ) ;
#105223=ORIENTED_EDGE ( 'NONE', *, *, #123966, .T. ) ;
#105408=AXIS2_PLACEMENT_3D ( 'NONE', #100238, #11257, #38582 ) ;
#105691=TOROIDAL_SURFACE ( 'NONE', #34659, 1.500000000000001776, 0.5000000000000000000 ) ;
#105920=AXIS2_PLACEMENT_3D ( 'NONE', #107122, #151664, #73842 ) ;
#105947=DIRECTION ( 'NONE',  ( -1.734723475976805122E-15, 0.1033298494363120712, 0.9946471445771455366 ) ) ;
#105951=AXIS2_PLACEMENT_3D ( 'NONE', #140381, #113020, #142369 ) ;
#106136=ADVANCED_FACE ( 'NONE', ( #146071 ), #144080, .T. ) ;
#106138=FACE_OUTER_BOUND ( 'NONE', #29163, .T. ) ;
#106320=DIRECTION ( 'NONE',  ( -1.000000000000000000, 0.000000000000000000, 0.000000000000000000 ) ) ;
#106434=EDGE_CURVE ( 'NONE', #183542, #87358, #4504, .T. ) ;
#106495=ORIENTED_EDGE ( 'NONE', *, *, #129926, .F. ) ;
#106967=EDGE_CURVE ( 'NONE', #87616, #66950, #175563, .T. ) ;
#106968=CARTESIAN_POINT ( 'NONE',  ( -4.500000000000001776, -139.5000000000000000, 22.27940468532398910 ) ) ;
#107122=CARTESIAN_POINT ( 'NONE',  ( -4.500000000000000888, -139.5000000000000000, 21.32407087589996308 ) ) ;
#107398=DIRECTION ( 'NONE',  ( -7.774220206137126725E-15, -0.8283630648959139364, 0.5601916035752839695 ) ) ;
#107481=ADVANCED_BREP_SHAPE_REPRESENTATION ( '', ( #5735, #82054 ), #188624 ) ;
#108348=AXIS2_PLACEMENT_3D ( 'NONE', #156729, #17217, #3036 ) ;
#108427=EDGE_LOOP ( 'NONE', ( #16488, #148216, #19213, #68079 ) ) ;
#108874=SPHERICAL_SURFACE ( 'NONE', #133892, 0.5000000000000000000 ) ;
#108990=ORIENTED_EDGE ( 'NONE', *, *, #78055, .F. ) ;
#109056=LINE ( 'NONE', #111043, #145153 ) ;
#109304=CARTESIAN_POINT ( 'NONE',  ( 5.000000000000000000, -126.1226662136678556, 8.481152457036387204 ) ) ;
#109394=CARTESIAN_POINT ( 'NONE',  ( 4.500000000000000888, -120.6140767358124180, 14.26817184396703198 ) ) ;
#109414=CARTESIAN_POINT ( 'NONE',  ( 4.500000000000000888, -139.5000000000000000, 21.82407087589996664 ) ) ;
#109420=ORIENTED_EDGE ( 'NONE', *, *, #18488, .T. ) ;
#109611=ADVANCED_FACE ( 'NONE', ( #183391 ), #93336, .F. ) ;
#109644=EDGE_CURVE ( 'NONE', #65926, #66950, #120703, .T. ) ;
#109893=DIRECTION ( 'NONE',  ( 0.000000000000000000, 0.000000000000000000, -1.000000000000000000 ) ) ;
#110318=EDGE_CURVE ( 'NONE', #123524, #80629, #152756, .T. ) ;
#110546=CARTESIAN_POINT ( 'NONE',  ( 4.500000000000000888, -126.1226662136678272, 8.481152457036385428 ) ) ;
#110819=AXIS2_PLACEMENT_3D ( 'NONE', #140487, #136517, #169835 ) ;
#111043=CARTESIAN_POINT ( 'NONE',  ( 5.000000000000000000, -130.0000000000000000, 12.99999999999999822 ) ) ;
#111198=( NAMED_UNIT ( * ) SI_UNIT ( $, .STERADIAN. ) SOLID_ANGLE_UNIT ( ) );
#111384=AXIS2_PLACEMENT_3D ( 'NONE', #68875, #161886, #158880 ) ;
#111627=CARTESIAN_POINT ( 'NONE',  ( -5.000000000000000000, -126.1226662136678272, 8.481152457036387204 ) ) ;
#111759=CARTESIAN_POINT ( 'NONE',  ( 4.500000000000000888, -139.5000000000000000, 13.35010376910484275 ) ) ;
#111989=ORIENTED_EDGE ( 'NONE', *, *, #2914, .T. ) ;
#111998=CIRCLE ( 'NONE', #47498, 0.5000000000000004441 ) ;
#112279=AXIS2_PLACEMENT_3D ( 'NONE', #122224, #30227, #35196 ) ;
#112421=AXIS2_PLACEMENT_3D ( 'NONE', #106968, #168642, #30141 ) ;
#112636=UNCERTAINTY_MEASURE_WITH_UNIT (LENGTH_MEASURE( 1.000000000000000082E-05 ), #14220, 'distance_accuracy_value', 'NONE');
#112832=ORIENTED_EDGE ( 'NONE', *, *, #10604, .F. ) ;
#112949=ORIENTED_EDGE ( 'NONE', *, *, #133407, .F. ) ;
#113020=DIRECTION ( 'NONE',  ( 0.000000000000000000, 0.9396926207859095381, -0.3420201433256656043 ) ) ;
#113377=DIRECTION ( 'NONE',  ( 0.000000000000000000, 0.000000000000000000, 1.000000000000000000 ) ) ;
#113385=CARTESIAN_POINT ( 'NONE',  ( -4.500000000000000888, -139.5000000000000000, 21.32407087589995953 ) ) ;
#113474=EDGE_CURVE ( 'NONE', #187814, #72196, #23746, .T. ) ;
#113718=EDGE_CURVE ( 'NONE', #84042, #123524, #150076, .T. ) ;
#113818=ORIENTED_EDGE ( 'NONE', *, *, #113474, .F. ) ;
#114038=ORIENTED_EDGE ( 'NONE', *, *, #168074, .F. ) ;
#114084=CARTESIAN_POINT ( 'NONE',  ( 4.500000000000000888, -126.1226662136678272, 7.981152457036389869 ) ) ;
#114103=DIRECTION ( 'NONE',  ( -1.000000000000000000, 0.000000000000000000, 6.938893903907234689E-15 ) ) ;
#114117=FACE_OUTER_BOUND ( 'NONE', #179899, .T. ) ;
#114395=COLOUR_RGB ( '', 0.09019608, 0.27058824, 0.51372549) ;
#114638=CARTESIAN_POINT ( 'NONE',  ( 4.500000000000000888, -139.5000000000000000, 21.32407087589996664 ) ) ;
#114650=DIRECTION ( 'NONE',  ( 0.000000000000000000, 0.000000000000000000, 1.000000000000000000 ) ) ;
#114733=DIRECTION ( 'NONE',  ( 0.000000000000000000, 0.000000000000000000, -1.000000000000000000 ) ) ;
#115618=CARTESIAN_POINT ( 'NONE',  ( 5.000000000000000000, -125.7396439921083555, 8.159758652193112027 ) ) ;
#116298=VECTOR ( 'NONE', #199327, 1000.000000000000000 ) ;
#116767=ORIENTED_EDGE ( 'NONE', *, *, #599, .F. ) ;
#116810=EDGE_CURVE ( 'NONE', #77030, #146728, #125938, .T. ) ;
#117016=CARTESIAN_POINT ( 'NONE',  ( 4.500000000000000888, -120.9454340326537505, 15.08688922109887187 ) ) ;
#117206=ORIENTED_EDGE ( 'NONE', *, *, #68789, .F. ) ;
#117570=EDGE_CURVE ( 'NONE', #72196, #37464, #164644, .T. ) ;
#117583=ORIENTED_EDGE ( 'NONE', *, *, #131422, .T. ) ;
#117593=AXIS2_PLACEMENT_3D ( 'NONE', #34819, #95490, #43297 ) ;
#117906=AXIS2_PLACEMENT_3D ( 'NONE', #174078, #83034, #6194 ) ;
#118219=AXIS2_PLACEMENT_3D ( 'NONE', #183273, #97927, #67613 ) ;
#118352=EDGE_CURVE ( 'NONE', #87358, #42462, #172614, .T. ) ;
#118669=CIRCLE ( 'NONE', #183174, 0.5000000000000012212 ) ;
#118796=DIRECTION ( 'NONE',  ( 0.000000000000000000, -0.5601916035752839695, -0.8283630648959138254 ) ) ;
#119531=FACE_OUTER_BOUND ( 'NONE', #3292, .T. ) ;
#119893=DIRECTION ( 'NONE',  ( 1.000000000000000000, 0.000000000000000000, -0.000000000000000000 ) ) ;
#120161=DIRECTION ( 'NONE',  ( -1.000000000000000000, 0.000000000000000000, 0.000000000000000000 ) ) ;
#120400=DIRECTION ( 'NONE',  ( 0.000000000000000000, 0.000000000000000000, 1.000000000000000000 ) ) ;
#120481=LINE ( 'NONE', #43658, #116298 ) ;
#120499=CARTESIAN_POINT ( 'NONE',  ( 4.500000000000000888, -130.0000000000000000, 13.99999999999999822 ) ) ;
#120505=DIRECTION ( 'NONE',  ( -1.000000000000000000, -0.000000000000000000, 0.000000000000000000 ) ) ;
#120669=DIRECTION ( 'NONE',  ( 0.000000000000000000, 0.000000000000000000, -1.000000000000000000 ) ) ;
#120703=LINE ( 'NONE', #124680, #42957 ) ;
#121112=CARTESIAN_POINT ( 'NONE',  ( 4.500000000000000888, -120.9970989573719038, 14.58956564881029827 ) ) ;
#121277=EDGE_CURVE ( 'NONE', #186287, #152202, #142091, .T. ) ;
#121849=ORIENTED_EDGE ( 'NONE', *, *, #148013, .F. ) ;
#121879=ORIENTED_EDGE ( 'NONE', *, *, #183827, .F. ) ;
#122224=CARTESIAN_POINT ( 'NONE',  ( -4.500000000000001776, -139.8289899283371653, 13.46984631039293845 ) ) ;
#122388=SURFACE_SIDE_STYLE ('',( #124380 ) ) ;
#123330=ADVANCED_FACE ( 'NONE', ( #94218 ), #15407, .T. ) ;
#123373=FILL_AREA_STYLE ('',( #156723 ) ) ;
#123524=VERTEX_POINT ( 'NONE', #109394 ) ;
#123555=DIRECTION ( 'NONE',  ( -6.938893903907222067E-15, 0.000000000000000000, -1.000000000000000000 ) ) ;
#123613=ORIENTED_EDGE ( 'NONE', *, *, #50743, .F. ) ;
#123966=EDGE_CURVE ( 'NONE', #183542, #84042, #132157, .T. ) ;
#124030=FACE_OUTER_BOUND ( 'NONE', #11186, .T. ) ;
#124042=CIRCLE ( 'NONE', #50180, 0.5000000000000004441 ) ;
#124181=APPLICATION_CONTEXT ( 'automotive_design' ) ;
#124380=SURFACE_STYLE_FILL_AREA ( #123373 ) ;
#124482=FACE_BOUND ( 'NONE', #24883, .T. ) ;
#124680=CARTESIAN_POINT ( 'NONE',  ( -5.000000000000000000, -139.5000000000000000, 22.27940468532398910 ) ) ;
#124778=DIRECTION ( 'NONE',  ( 0.000000000000000000, 0.000000000000000000, 1.000000000000000000 ) ) ;
#124896=CARTESIAN_POINT ( 'NONE',  ( -5.000000000000000000, -120.9970989573719038, 14.58956564881029472 ) ) ;
#124967=VERTEX_POINT ( 'NONE', #22375 ) ;
#124993=AXIS2_PLACEMENT_3D ( 'NONE', #94697, #185729, #50205 ) ;
#125120=AXIS2_PLACEMENT_3D ( 'NONE', #177302, #87269, #10443 ) ;
#125539=ORIENTED_EDGE ( 'NONE', *, *, #186126, .F. ) ;
#125845=SHAPE_REPRESENTATION ( 'Switch', ( #82054 ), #188624 ) ;
#125938=CIRCLE ( 'NONE', #54933, 1.500000000000001332 ) ;
#126119=ORIENTED_EDGE ( 'NONE', *, *, #110318, .F. ) ;
#126210=FACE_OUTER_BOUND ( 'NONE', #101443, .T. ) ;
#126547=CARTESIAN_POINT ( 'NONE',  ( 4.500000000000000888, -130.0000000000000000, 15.50000000000000000 ) ) ;
#127243=AXIS2_PLACEMENT_3D ( 'NONE', #178074, #191232, #9224 ) ;
#127276=CIRCLE ( 'NONE', #72330, 40.49999999999999289 ) ;
#127342=EDGE_LOOP ( 'NONE', ( #14468, #186235, #91190, #50472 ) ) ;
#129093=DIRECTION ( 'NONE',  ( 0.000000000000000000, 0.000000000000000000, -1.000000000000000000 ) ) ;
#129135=ADVANCED_FACE ( 'NONE', ( #175174 ), #6269, .T. ) ;
#129477=LINE ( 'NONE', #37485, #164537 ) ;
#129482=APPLICATION_CONTEXT ( 'automotive_design' ) ;
#129514=ORIENTED_EDGE ( 'NONE', *, *, #189089, .T. ) ;
#129600=ORIENTED_EDGE ( 'NONE', *, *, #68789, .T. ) ;
#129763=CYLINDRICAL_SURFACE ( 'NONE', #101748, 0.5000000000000006661 ) ;
#129817=CYLINDRICAL_SURFACE ( 'NONE', #5599, 0.5000000000000004441 ) ;
#129926=EDGE_CURVE ( 'NONE', #198944, #35288, #164509, .T. ) ;
#130190=DIRECTION ( 'NONE',  ( -1.000000000000000000, 0.000000000000000000, 0.000000000000000000 ) ) ;
#130569=SPHERICAL_SURFACE ( 'NONE', #182921, 0.5000000000000000000 ) ;
#130653=CARTESIAN_POINT ( 'NONE',  ( -5.000000000000000000, -130.0000000000000000, 13.99999999999999822 ) ) ;
#130787=AXIS2_PLACEMENT_3D ( 'NONE', #5395, #20571, #124778 ) ;
#130805=DIRECTION ( 'NONE',  ( 1.000000000000000000, 0.000000000000000000, -0.000000000000000000 ) ) ;
#131422=EDGE_CURVE ( 'NONE', #90572, #185765, #46278, .T. ) ;
#131523=AXIS2_PLACEMENT_3D ( 'NONE', #48868, #199571, #15549 ) ;
#131667=CARTESIAN_POINT ( 'NONE',  ( 4.500000000000000888, -130.0000000000000000, 13.99999999999999822 ) ) ;
#132157=CIRCLE ( 'NONE', #25528, 0.5000000000000004441 ) ;
#132178=DIRECTION ( 'NONE',  ( -1.734723475976805517E-15, 0.3420201433256828127, 0.9396926207859033209 ) ) ;
#132257=LINE ( 'NONE', #54419, #76495 ) ;
#132862=ORIENTED_EDGE ( 'NONE', *, *, #18488, .F. ) ;
#133249=DIRECTION ( 'NONE',  ( -0.000000000000000000, -0.9396926207859095381, 0.3420201433256656043 ) ) ;
#133299=CARTESIAN_POINT ( 'NONE',  ( -4.500000000000000888, -126.1226662136678272, 8.481152457036387204 ) ) ;
#133302=EDGE_CURVE ( 'NONE', #34377, #90572, #124042, .T. ) ;
#133375=LINE ( 'NONE', #150559, #11532 ) ;
#133407=EDGE_CURVE ( 'NONE', #94299, #124967, #133375, .T. ) ;
#133598=ORIENTED_EDGE ( 'NONE', *, *, #2819, .F. ) ;
#133892=AXIS2_PLACEMENT_3D ( 'NONE', #16873, #153388, #170554 ) ;
#133910=DIRECTION ( 'NONE',  ( 1.000000000000000000, -0.000000000000000000, -0.000000000000000000 ) ) ;
#133958=CARTESIAN_POINT ( 'NONE',  ( 4.500000000000000888, -139.5000000000000000, 21.32407087589995953 ) ) ;
#134108=DIRECTION ( 'NONE',  ( -1.000000000000000000, 0.000000000000000000, 0.000000000000000000 ) ) ;
#134138=ORIENTED_EDGE ( 'NONE', *, *, #121277, .F. ) ;
#134292=EDGE_CURVE ( 'NONE', #87243, #185765, #40522, .T. ) ;
#134560=DIRECTION ( 'NONE',  ( -1.000000000000000000, -0.000000000000000000, -0.000000000000000000 ) ) ;
#134963=CARTESIAN_POINT ( 'NONE',  ( 4.500000000000000888, -125.7396439921083555, 8.159758652193113804 ) ) ;
#135522=ORIENTED_EDGE ( 'NONE', *, *, #74471, .T. ) ;
#135864=DIRECTION ( 'NONE',  ( -1.000000000000000000, -0.000000000000000000, -0.000000000000000000 ) ) ;
#136057=DIRECTION ( 'NONE',  ( 0.000000000000000000, -1.734723475976807489E-15, 1.000000000000000000 ) ) ;
#136515=ORIENTED_EDGE ( 'NONE', *, *, #137830, .F. ) ;
#136517=DIRECTION ( 'NONE',  ( 1.186620743768021534E-15, -0.9396926207859040980, 0.3420201433256805368 ) ) ;
#136742=VECTOR ( 'NONE', #133910, 1000.000000000000000 ) ;
#136873=DIRECTION ( 'NONE',  ( -0.000000000000000000, -0.000000000000000000, 1.000000000000000000 ) ) ;
#137265=DIRECTION ( 'NONE',  ( -1.000000000000000000, -0.000000000000000000, -0.000000000000000000 ) ) ;
#137340=ORIENTED_EDGE ( 'NONE', *, *, #98904, .T. ) ;
#137663=PLANE ( 'NONE',  #166405 ) ;
#137676=CIRCLE ( 'NONE', #50504, 0.5000000000000004441 ) ;
#137746=CARTESIAN_POINT ( 'NONE',  ( -4.500000000000001776, -120.9970989573719038, 14.58956564881029827 ) ) ;
#137830=EDGE_CURVE ( 'NONE', #123524, #146762, #8918, .T. ) ;
#137835=AXIS2_PLACEMENT_3D ( 'NONE', #92701, #1694, #18872 ) ;
#137913=SPHERICAL_SURFACE ( 'NONE', #8263, 0.5000000000000000000 ) ;
#138261=LINE ( 'NONE', #28132, #69705 ) ;
#138616=ADVANCED_FACE ( 'NONE', ( #93701 ), #108874, .T. ) ;
#139720=DIRECTION ( 'NONE',  ( 0.000000000000000000, 1.000000000000000000, 0.000000000000000000 ) ) ;
#139747=AXIS2_PLACEMENT_3D ( 'NONE', #185124, #152791, #91103 ) ;
#140120=ORIENTED_EDGE ( 'NONE', *, *, #174667, .T. ) ;
#140361=VECTOR ( 'NONE', #134108, 1000.000000000000000 ) ;
#140381=CARTESIAN_POINT ( 'NONE',  ( 4.500000000000000888, -132.8113331068338425, 10.91562811307058389 ) ) ;
#140467=CIRCLE ( 'NONE', #130787, 0.5000000000000004441 ) ;
#140487=CARTESIAN_POINT ( 'NONE',  ( 4.500000000000000888, -139.5000000000000000, 13.35010376910484275 ) ) ;
#140518=ORIENTED_EDGE ( 'NONE', *, *, #164973, .T. ) ;
#140551=EDGE_LOOP ( 'NONE', ( #152879, #125539, #146560, #113818, #35577 ) ) ;
#140725=CARTESIAN_POINT ( 'NONE',  ( 4.500000000000000888, -120.9970989573719038, 14.58956564881029649 ) ) ;
#141384=CARTESIAN_POINT ( 'NONE',  ( -4.500000000000001776, -116.8122400552013431, 54.87277500418469600 ) ) ;
#141440=DIRECTION ( 'NONE',  ( 0.000000000000000000, 0.000000000000000000, 1.000000000000000000 ) ) ;
#141847=DIRECTION ( 'NONE',  ( -1.000000000000000000, -0.000000000000000000, -0.000000000000000000 ) ) ;
#141875=DIRECTION ( 'NONE',  ( 0.000000000000000000, 0.7660444431189601389, -0.6427876096865606792 ) ) ;
#141961=DIRECTION ( 'NONE',  ( 0.000000000000000000, -0.6427876096865404731, -0.7660444431189771253 ) ) ;
#142091=CIRCLE ( 'NONE', #193797, 1.000000000000000888 ) ;
#142191=DIRECTION ( 'NONE',  ( -1.000000000000000000, -0.000000000000000000, 0.000000000000000000 ) ) ;
#142369=DIRECTION ( 'NONE',  ( 0.000000000000000000, 0.3420201433256804813, 0.9396926207859040980 ) ) ;
#142437=EDGE_CURVE ( 'NONE', #39277, #12274, #163444, .T. ) ;
#142864=DIRECTION ( 'NONE',  ( 0.000000000000000000, -0.9396926207859049862, 0.3420201433256783163 ) ) ;
#143000=ORIENTED_EDGE ( 'NONE', *, *, #2819, .T. ) ;
#143028=CARTESIAN_POINT ( 'NONE',  ( -4.500000000000001776, -140.0000000000000000, 21.32407087589996308 ) ) ;
#143178=CARTESIAN_POINT ( 'NONE',  ( -4.500000000000001776, -130.0000000000000000, 13.99999999999999822 ) ) ;
#143331=EDGE_LOOP ( 'NONE', ( #162701, #24413, #31777, #13630 ) ) ;
#143416=COLOUR_RGB ( '', 0.09019608, 0.27058824, 0.51372549) ;
#143427=VERTEX_POINT ( 'NONE', #88765 ) ;
#143440=VECTOR ( 'NONE', #15492, 1000.000000000000114 ) ;
#143450=FACE_OUTER_BOUND ( 'NONE', #46562, .T. ) ;
#143497=ORIENTED_EDGE ( 'NONE', *, *, #47680, .T. ) ;
#144056=AXIS2_PLACEMENT_3D ( 'NONE', #114638, #130805, #145972 ) ;
#144080=SPHERICAL_SURFACE ( 'NONE', #59375, 0.5000000000000000000 ) ;
#144207=CIRCLE ( 'NONE', #170061, 0.5000000000000006661 ) ;
#144774=EDGE_CURVE ( 'NONE', #87243, #34377, #183768, .T. ) ;
#144857=DIRECTION ( 'NONE',  ( 0.000000000000000000, -0.3420201433256828127, -0.9396926207859033209 ) ) ;
#145074=DIRECTION ( 'NONE',  ( -0.000000000000000000, -0.9946471445771456477, 0.1033298494363113634 ) ) ;
#145106=DIRECTION ( 'NONE',  ( -0.000000000000000000, -0.9396926207858838920, 0.3420201433257362145 ) ) ;
#145153=VECTOR ( 'NONE', #19050, 1000.000000000000000 ) ;
#145274=CYLINDRICAL_SURFACE ( 'NONE', #95957, 0.5000000000000017764 ) ;
#145468=EDGE_CURVE ( 'NONE', #124967, #197216, #101702, .T. ) ;
#145715=DIRECTION ( 'NONE',  ( -1.000000000000000000, -0.000000000000000000, 0.000000000000000000 ) ) ;
#145972=DIRECTION ( 'NONE',  ( 0.000000000000000000, 0.000000000000000000, -1.000000000000000000 ) ) ;
#146071=FACE_OUTER_BOUND ( 'NONE', #13394, .T. ) ;
#146092=ORIENTED_EDGE ( 'NONE', *, *, #144774, .F. ) ;
#146270=CARTESIAN_POINT ( 'NONE',  ( 4.500000000000000888, -99.43240762267087973, 40.28936402012540441 ) ) ;
#146275=PRODUCT_CONTEXT ( 'NONE', #124181, 'mechanical' ) ;
#146491=ADVANCED_FACE ( 'NONE', ( #378 ), #137913, .T. ) ;
#146560=ORIENTED_EDGE ( 'NONE', *, *, #50546, .F. ) ;
#146728=VERTEX_POINT ( 'NONE', #88430 ) ;
#146762=VERTEX_POINT ( 'NONE', #134963 ) ;
#147019=CARTESIAN_POINT ( 'NONE',  ( 5.000000000000000000, -139.5000000000000000, 21.32407087589996308 ) ) ;
#147675=DIRECTION ( 'NONE',  ( 1.000000000000000000, -0.000000000000000000, -0.000000000000000000 ) ) ;
#147960=DIRECTION ( 'NONE',  ( 0.000000000000000000, 0.000000000000000000, 1.000000000000000000 ) ) ;
#148013=EDGE_CURVE ( 'NONE', #146762, #37464, #169766, .T. ) ;
#148216=ORIENTED_EDGE ( 'NONE', *, *, #95661, .F. ) ;
#148445=DIRECTION ( 'NONE',  ( 0.000000000000000000, 0.6427876096865403621, 0.7660444431189770143 ) ) ;
#148714=ORIENTED_EDGE ( 'NONE', *, *, #92523, .T. ) ;
#149965=DIRECTION ( 'NONE',  ( -0.000000000000000000, -0.9396926207859095381, 0.3420201433256656043 ) ) ;
#150076=LINE ( 'NONE', #72234, #136742 ) ;
#150249=CARTESIAN_POINT ( 'NONE',  ( 4.500000000000000888, -116.8122400552013431, 54.87277500418469600 ) ) ;
#150452=LINE ( 'NONE', #11948, #170341 ) ;
#150559=CARTESIAN_POINT ( 'NONE',  ( 5.000000000000000000, -139.2199041982123617, 21.73825240834792538 ) ) ;
#150773=ORIENTED_EDGE ( 'NONE', *, *, #133407, .T. ) ;
#150868=FACE_OUTER_BOUND ( 'NONE', #154550, .T. ) ;
#151664=DIRECTION ( 'NONE',  ( -0.000000000000000000, -1.000000000000000000, 0.000000000000000000 ) ) ;
#151687=EDGE_CURVE ( 'NONE', #197216, #185765, #92395, .T. ) ;
#151851=CARTESIAN_POINT ( 'NONE',  ( -5.000000000000000000, -116.8122400552013431, 54.87277500418469600 ) ) ;
#151994=ORIENTED_EDGE ( 'NONE', *, *, #78055, .T. ) ;
#152202=VERTEX_POINT ( 'NONE', #189511 ) ;
#152756=CIRCLE ( 'NONE', #139747, 0.5000000000000004441 ) ;
#152791=DIRECTION ( 'NONE',  ( 1.000000000000000000, -0.000000000000000000, 0.000000000000000000 ) ) ;
#152794=ORIENTED_EDGE ( 'NONE', *, *, #113718, .F. ) ;
#152879=ORIENTED_EDGE ( 'NONE', *, *, #198827, .F. ) ;
#153026=CARTESIAN_POINT ( 'NONE',  ( 5.000000000000000000, -130.0000000000000000, 13.99999999999999822 ) ) ;
#153032=DIRECTION ( 'NONE',  ( 0.000000000000000000, 1.000000000000000000, 0.000000000000000000 ) ) ;
#153051=DIRECTION ( 'NONE',  ( 0.000000000000000000, 0.000000000000000000, 1.000000000000000000 ) ) ;
#153126=CIRCLE ( 'NONE', #156314, 1.500000000000001332 ) ;
#153271=CIRCLE ( 'NONE', #24115, 0.5000000000000004441 ) ;
#153388=DIRECTION ( 'NONE',  ( 0.000000000000000000, 1.000000000000000000, -0.000000000000000000 ) ) ;
#153423=EDGE_LOOP ( 'NONE', ( #187319, #70935, #42011, #171046 ) ) ;
#153513=AXIS2_PLACEMENT_3D ( 'NONE', #161896, #23392, #51718 ) ;
#154234=DIRECTION ( 'NONE',  ( 0.000000000000000000, 0.000000000000000000, 1.000000000000000000 ) ) ;
#154421=ORIENTED_EDGE ( 'NONE', *, *, #182367, .T. ) ;
#154496=ORIENTED_EDGE ( 'NONE', *, *, #169612, .F. ) ;
#154550=EDGE_LOOP ( 'NONE', ( #151994, #196475, #63974, #102717 ) ) ;
#155047=FACE_OUTER_BOUND ( 'NONE', #81459, .T. ) ;
#155079=PRODUCT ( 'Switch', 'Switch', '', ( #146275 ) ) ;
#155639=CARTESIAN_POINT ( 'NONE',  ( -4.500000000000001776, -139.5000000000000000, 21.82407087589996308 ) ) ;
#155898=CIRCLE ( 'NONE', #52697, 0.5000000000000004441 ) ;
#156016=DIRECTION ( 'NONE',  ( -1.387778780781444413E-14, 0.000000000000000000, 1.000000000000000000 ) ) ;
#156147=FACE_OUTER_BOUND ( 'NONE', #92434, .T. ) ;
#156264=FILL_AREA_STYLE ('',( #15773 ) ) ;
#156314=AXIS2_PLACEMENT_3D ( 'NONE', #89075, #166929, #120400 ) ;
#156544=EDGE_LOOP ( 'NONE', ( #23582, #183356, #39762 ) ) ;
#156556=CYLINDRICAL_SURFACE ( 'NONE', #105951, 0.5000000000000037748 ) ;
#156723=FILL_AREA_STYLE_COLOUR ( '', #143416 ) ;
#156729=CARTESIAN_POINT ( 'NONE',  ( 4.500000000000000888, -130.0000000000000000, 13.99999999999999822 ) ) ;
#157403=DIRECTION ( 'NONE',  ( 1.000000000000000000, 0.000000000000000000, -0.000000000000000000 ) ) ;
#157409=ORIENTED_EDGE ( 'NONE', *, *, #100701, .T. ) ;
#157548=EDGE_CURVE ( 'NONE', #17604, #146728, #140467, .T. ) ;
#157557=DIRECTION ( 'NONE',  ( 0.000000000000000000, 0.000000000000000000, 1.000000000000000000 ) ) ;
#157612=FACE_OUTER_BOUND ( 'NONE', #163117, .T. ) ;
#157679=CARTESIAN_POINT ( 'NONE',  ( -4.500000000000001776, -126.1226662136678272, 8.481152457036383652 ) ) ;
#158431=CIRCLE ( 'NONE', #184283, 39.99999999999999289 ) ;
#158880=DIRECTION ( 'NONE',  ( 0.000000000000000000, 0.000000000000000000, 1.000000000000000000 ) ) ;
#159879=VECTOR ( 'NONE', #104212, 1000.000000000000000 ) ;
#160083=ORIENTED_EDGE ( 'NONE', *, *, #134292, .T. ) ;
#160467=ORIENTED_EDGE ( 'NONE', *, *, #164973, .F. ) ;
#161284=CARTESIAN_POINT ( 'NONE',  ( 4.500000000000000888, -126.1226662136678272, 8.481152457036383652 ) ) ;
#161701=ADVANCED_FACE ( 'NONE', ( #119531 ), #37642, .T. ) ;
#161714=ORIENTED_EDGE ( 'NONE', *, *, #20610, .F. ) ;
#161836=ADVANCED_FACE ( 'NONE', ( #150868 ), #2002, .T. ) ;
#161886=DIRECTION ( 'NONE',  ( -1.000000000000000000, -0.000000000000000000, 0.000000000000000000 ) ) ;
#161896=CARTESIAN_POINT ( 'NONE',  ( 4.500000000000000888, -139.5000000000000000, 21.32407087589996308 ) ) ;
#162167=ORIENTED_EDGE ( 'NONE', *, *, #183827, .T. ) ;
#162701=ORIENTED_EDGE ( 'NONE', *, *, #599, .T. ) ;
#163117=EDGE_LOOP ( 'NONE', ( #88851, #66078, #194434, #199279 ) ) ;
#163302=ADVANCED_FACE ( 'NONE', ( #2126 ), #91135, .T. ) ;
#163444=LINE ( 'NONE', #26940, #140361 ) ;
#163725=ORIENTED_EDGE ( 'NONE', *, *, #187343, .T. ) ;
#164046=DIRECTION ( 'NONE',  ( 0.000000000000000000, 0.000000000000000000, 1.000000000000000000 ) ) ;
#164479=ORIENTED_EDGE ( 'NONE', *, *, #50912, .F. ) ;
#164509=CIRCLE ( 'NONE', #77300, 1.500000000000001332 ) ;
#164537=VECTOR ( 'NONE', #147675, 1000.000000000000000 ) ;
#164644=CIRCLE ( 'NONE', #9776, 0.5000000000000004441 ) ;
#164973=EDGE_CURVE ( 'NONE', #71610, #94299, #137676, .T. ) ;
#165342=ORIENTED_EDGE ( 'NONE', *, *, #157548, .F. ) ;
#165368=CARTESIAN_POINT ( 'NONE',  ( -4.500000000000001776, -139.5000000000000000, 13.35010376910484098 ) ) ;
#165475=ORIENTED_EDGE ( 'NONE', *, *, #198827, .T. ) ;
#165889=LINE ( 'NONE', #60666, #83121 ) ;
#166117=MECHANICAL_DESIGN_GEOMETRIC_PRESENTATION_REPRESENTATION('',(#4699),#198430);
#166125=STYLED_ITEM ( 'NONE', ( #199247 ), #107481 ) ;
#166148=CIRCLE ( 'NONE', #40269, 0.5000000000000004441 ) ;
#166405=AXIS2_PLACEMENT_3D ( 'NONE', #151851, #120505, #59827 ) ;
#166626=EDGE_LOOP ( 'NONE', ( #129600, #71174, #70645, #71199 ) ) ;
#166929=DIRECTION ( 'NONE',  ( 1.000000000000000000, 0.000000000000000000, -0.000000000000000000 ) ) ;
#167527=EDGE_CURVE ( 'NONE', #187814, #37464, #99118, .T. ) ;
#168074=EDGE_CURVE ( 'NONE', #123524, #49927, #173330, .T. ) ;
#168170=CARTESIAN_POINT ( 'NONE',  ( 5.000000000000000000, -99.43240762267087973, 40.28936402012540441 ) ) ;
#168190=EDGE_CURVE ( 'NONE', #87243, #124967, #86149, .T. ) ;
#168329=DIRECTION ( 'NONE',  ( 1.000000000000000000, 0.000000000000000000, -0.000000000000000000 ) ) ;
#168642=DIRECTION ( 'NONE',  ( 0.000000000000000000, 0.000000000000000000, 1.000000000000000000 ) ) ;
#168645=DIRECTION ( 'NONE',  ( 0.000000000000000000, 0.000000000000000000, 1.000000000000000000 ) ) ;
#169612=EDGE_CURVE ( 'NONE', #66950, #87358, #183023, .T. ) ;
#169766=CIRCLE ( 'NONE', #98730, 0.4999999999999945044 ) ;
#169835=DIRECTION ( 'NONE',  ( 0.000000000000000000, -0.3420201433256828127, -0.9396926207859033209 ) ) ;
#169895=( NAMED_UNIT ( * ) PLANE_ANGLE_UNIT ( ) SI_UNIT ( $, .RADIAN. ) );
#170061=AXIS2_PLACEMENT_3D ( 'NONE', #5989, #50527, #17200 ) ;
#170200=SPHERICAL_SURFACE ( 'NONE', #88735, 0.5000000000000000000 ) ;
#170219=FACE_OUTER_BOUND ( 'NONE', #56771, .T. ) ;
#170248=CARTESIAN_POINT ( 'NONE',  ( 4.500000000000000888, -126.1226662136678272, 8.481152457036388981 ) ) ;
#170341=VECTOR ( 'NONE', #148445, 1000.000000000000114 ) ;
#170444=( LENGTH_UNIT ( ) NAMED_UNIT ( * ) SI_UNIT ( .MILLI., .METRE. ) );
#170554=DIRECTION ( 'NONE',  ( 6.938893903907222067E-15, 0.000000000000000000, 1.000000000000000000 ) ) ;
#171046=ORIENTED_EDGE ( 'NONE', *, *, #134292, .F. ) ;
#171353=ADVANCED_FACE ( 'NONE', ( #25624 ), #178295, .T. ) ;
#171637=CARTESIAN_POINT ( 'NONE',  ( -4.500000000000001776, -120.6140767358124180, 14.26817184396703198 ) ) ;
#172508=ADVANCED_FACE ( 'NONE', ( #20936 ), #145274, .T. ) ;
#172614=LINE ( 'NONE', #49270, #196981 ) ;
#172699=AXIS2_PLACEMENT_3D ( 'NONE', #51095, #188630, #98571 ) ;
#172705=ORIENTED_EDGE ( 'NONE', *, *, #73810, .T. ) ;
#173025=CARTESIAN_POINT ( 'NONE',  ( -4.500000000000001776, -139.2199041982123617, 21.73825240834792893 ) ) ;
#173330=CIRCLE ( 'NONE', #189496, 0.4999999999999972800 ) ;
#173731=CARTESIAN_POINT ( 'NONE',  ( 5.000000000000000000, -140.0000000000000000, 12.99999999999998224 ) ) ;
#174078=CARTESIAN_POINT ( 'NONE',  ( 5.000000000000000000, -120.9970989573719038, 14.58956564881029649 ) ) ;
#174230=CARTESIAN_POINT ( 'NONE',  ( -5.000000000000000000, -116.8122400552013431, 54.87277500418469600 ) ) ;
#174667=EDGE_CURVE ( 'NONE', #87616, #4972, #85327, .T. ) ;
#174806=ADVANCED_FACE ( 'NONE', ( #97484 ), #129817, .T. ) ;
#174836=CARTESIAN_POINT ( 'NONE',  ( -5.000000000000000888, -130.0000000000000000, 12.49999999999999645 ) ) ;
#175174=FACE_OUTER_BOUND ( 'NONE', #42047, .T. ) ;
#175563=CIRCLE ( 'NONE', #40036, 0.5000000000000004441 ) ;
#176516=AXIS2_PLACEMENT_3D ( 'NONE', #109304, #106320, #63808 ) ;
#176665=AXIS2_PLACEMENT_3D ( 'NONE', #161284, #145106, #53098 ) ;
#176970=AXIS2_PLACEMENT_3D ( 'NONE', #133299, #194990, #29129 ) ;
#177111=CYLINDRICAL_SURFACE ( 'NONE', #105408, 39.99999999999999289 ) ;
#177302=CARTESIAN_POINT ( 'NONE',  ( 4.500000000000000888, -139.5000000000000000, 54.87277500418469600 ) ) ;
#177443=DIRECTION ( 'NONE',  ( -1.734723475976805122E-15, 0.1033298494363120712, 0.9946471445771455366 ) ) ;
#177810=DIRECTION ( 'NONE',  ( -6.938893903907246521E-15, -0.000000000000000000, -1.000000000000000000 ) ) ;
#178074=CARTESIAN_POINT ( 'NONE',  ( 5.000000000000000000, -130.0000000000000000, 13.99999999999999822 ) ) ;
#178102=ORIENTED_EDGE ( 'NONE', *, *, #123966, .F. ) ;
#178295=CYLINDRICAL_SURFACE ( 'NONE', #125120, 0.5000000000000004441 ) ;
#178509=EDGE_LOOP ( 'NONE', ( #62487, #143000 ) ) ;
#179267=PRODUCT_DEFINITION_FORMATION_WITH_SPECIFIED_SOURCE ( 'ANY', '', #155079, .NOT_KNOWN. ) ;
#179746=CARTESIAN_POINT ( 'NONE',  ( -4.500000000000001776, -139.5000000000000000, 21.32407087589996308 ) ) ;
#179899=EDGE_LOOP ( 'NONE', ( #30328, #192191, #112949, #160467 ) ) ;
#180537=ORIENTED_EDGE ( 'NONE', *, *, #118352, .F. ) ;
#180856=ADVANCED_FACE ( 'NONE', ( #106138 ), #74821, .T. ) ;
#180869=FACE_OUTER_BOUND ( 'NONE', #108427, .T. ) ;
#181003=EDGE_CURVE ( 'NONE', #71610, #66950, #44589, .T. ) ;
#181382=ORIENTED_EDGE ( 'NONE', *, *, #187343, .F. ) ;
#181445=CARTESIAN_POINT ( 'NONE',  ( -4.500000000000001776, -125.9646863569935107, 7.891563605355330857 ) ) ;
#182190=DIRECTION ( 'NONE',  ( -1.000000000000000000, -0.000000000000000000, 0.000000000000000000 ) ) ;
#182367=EDGE_CURVE ( 'NONE', #187814, #39277, #132257, .T. ) ;
#182548=AXIS2_PLACEMENT_3D ( 'NONE', #98688, #157403, #83522 ) ;
#182921=AXIS2_PLACEMENT_3D ( 'NONE', #101230, #194275, #56756 ) ;
#183023=CIRCLE ( 'NONE', #95816, 40.49999999999999289 ) ;
#183174=AXIS2_PLACEMENT_3D ( 'NONE', #45746, #107398, #27629 ) ;
#183273=CARTESIAN_POINT ( 'NONE',  ( 5.000000000000000000, -140.0000000000000000, 22.27940468532398910 ) ) ;
#183356=ORIENTED_EDGE ( 'NONE', *, *, #10604, .T. ) ;
#183391=FACE_OUTER_BOUND ( 'NONE', #191155, .T. ) ;
#183501=ORIENTED_EDGE ( 'NONE', *, *, #181003, .T. ) ;
#183542=VERTEX_POINT ( 'NONE', #57428 ) ;
#183768=LINE ( 'NONE', #186768, #53338 ) ;
#183827=EDGE_CURVE ( 'NONE', #49235, #17604, #95970, .T. ) ;
#184133=CARTESIAN_POINT ( 'NONE',  ( 4.500000000000000888, -139.6710100716628631, 12.88025745871188654 ) ) ;
#184283=AXIS2_PLACEMENT_3D ( 'NONE', #141384, #34211, #157557 ) ;
#184302=ADVANCED_FACE ( 'NONE', ( #32046 ), #66811, .T. ) ;
#184460=ADVANCED_FACE ( 'NONE', ( #124030 ), #48214, .F. ) ;
#184623=PRESENTATION_STYLE_ASSIGNMENT (( #61266 ) ) ;
#185124=CARTESIAN_POINT ( 'NONE',  ( 4.500000000000000888, -120.9970989573719038, 14.58956564881030005 ) ) ;
#185215=EDGE_CURVE ( 'NONE', #4972, #12274, #111998, .T. ) ;
#185729=DIRECTION ( 'NONE',  ( -1.000000000000000000, -0.000000000000000000, -0.000000000000000000 ) ) ;
#185765=VERTEX_POINT ( 'NONE', #76311 ) ;
#186075=SURFACE_STYLE_USAGE ( .BOTH. , #122388 ) ;
#186126=EDGE_CURVE ( 'NONE', #146762, #1415, #85260, .T. ) ;
#186235=ORIENTED_EDGE ( 'NONE', *, *, #109644, .F. ) ;
#186287=VERTEX_POINT ( 'NONE', #70112 ) ;
#186768=CARTESIAN_POINT ( 'NONE',  ( 5.000000000000000000, -139.5000000000000000, 54.87277500418469600 ) ) ;
#187319=ORIENTED_EDGE ( 'NONE', *, *, #168190, .T. ) ;
#187343=EDGE_CURVE ( 'NONE', #87616, #71610, #92344, .T. ) ;
#187386=ADVANCED_FACE ( 'NONE', ( #143450 ), #17153, .F. ) ;
#187400=CARTESIAN_POINT ( 'NONE',  ( -4.500000000000001776, -130.0000000000000000, 13.99999999999999822 ) ) ;
#187814=VERTEX_POINT ( 'NONE', #1972 ) ;
#187906=DIRECTION ( 'NONE',  ( 0.000000000000000000, -0.6427876096865403621, -0.7660444431189770143 ) ) ;
#188483=EDGE_CURVE ( 'NONE', #4972, #65926, #192392, .T. ) ;
#188624=( GEOMETRIC_REPRESENTATION_CONTEXT ( 3 ) GLOBAL_UNCERTAINTY_ASSIGNED_CONTEXT ( ( #189501 ) ) GLOBAL_UNIT_ASSIGNED_CONTEXT ( ( #34369, #169895, #111198 ) ) REPRESENTATION_CONTEXT ( 'NONE', 'WORKASPACE' ) );
#188630=DIRECTION ( 'NONE',  ( 0.000000000000000000, 1.000000000000000000, 0.000000000000000000 ) ) ;
#188721=DIRECTION ( 'NONE',  ( 0.000000000000000000, 0.000000000000000000, 1.000000000000000000 ) ) ;
#188898=CARTESIAN_POINT ( 'NONE',  ( 5.000000000000000000, -120.0000000000000142, 14.99999999999998757 ) ) ;
#189089=EDGE_CURVE ( 'NONE', #49235, #152202, #138261, .T. ) ;
#189245=DIRECTION ( 'NONE',  ( 0.000000000000000000, 0.000000000000000000, -1.000000000000000000 ) ) ;
#189442=ORIENTED_EDGE ( 'NONE', *, *, #167527, .F. ) ;
#189496=AXIS2_PLACEMENT_3D ( 'NONE', #192630, #71284, #195649 ) ;
#189501=UNCERTAINTY_MEASURE_WITH_UNIT (LENGTH_MEASURE( 1.000000000000000082E-05 ), #34369, 'distance_accuracy_value', 'NONE');
#189511=CARTESIAN_POINT ( 'NONE',  ( -4.500000000000001776, -130.0000000000000000, 15.00000000000000000 ) ) ;
#190998=DIRECTION ( 'NONE',  ( 0.000000000000000000, 0.000000000000000000, 1.000000000000000000 ) ) ;
#191155=EDGE_LOOP ( 'NONE', ( #197771, #46137, #129514, #111989 ) ) ;
#191232=DIRECTION ( 'NONE',  ( -1.000000000000000000, -0.000000000000000000, 0.000000000000000000 ) ) ;
#191448=DIRECTION ( 'NONE',  ( -1.000000000000000000, 0.000000000000000000, 0.000000000000000000 ) ) ;
#191886=DIRECTION ( 'NONE',  ( 0.000000000000000000, 0.000000000000000000, 1.000000000000000000 ) ) ;
#191927=( GEOMETRIC_REPRESENTATION_CONTEXT ( 3 ) GLOBAL_UNCERTAINTY_ASSIGNED_CONTEXT ( ( #112636 ) ) GLOBAL_UNIT_ASSIGNED_CONTEXT ( ( #14220, #75889, #48553 ) ) REPRESENTATION_CONTEXT ( 'NONE', 'WORKASPACE' ) );
#191960=CARTESIAN_POINT ( 'NONE',  ( -4.500000000000001776, -139.5000000000000000, 13.35010376910484275 ) ) ;
#192191=ORIENTED_EDGE ( 'NONE', *, *, #145468, .F. ) ;
#192392=CIRCLE ( 'NONE', #27740, 0.4999999999999995559 ) ;
#192528=DIRECTION ( 'NONE',  ( 0.000000000000000000, 0.000000000000000000, 1.000000000000000000 ) ) ;
#192630=CARTESIAN_POINT ( 'NONE',  ( 4.500000000000000888, -120.9970989573719038, 14.58956564881029294 ) ) ;
#193049=ORIENTED_EDGE ( 'NONE', *, *, #58736, .T. ) ;
#193069=EDGE_CURVE ( 'NONE', #39277, #34377, #36610, .T. ) ;
#193349=DIRECTION ( 'NONE',  ( -1.000000000000000000, -0.000000000000000000, 0.000000000000000000 ) ) ;
#193375=DIRECTION ( 'NONE',  ( 0.000000000000000000, 0.000000000000000000, 1.000000000000000000 ) ) ;
#193532=DIRECTION ( 'NONE',  ( 0.000000000000000000, 0.000000000000000000, -1.000000000000000000 ) ) ;
#193797=AXIS2_PLACEMENT_3D ( 'NONE', #12697, #197703, #44019 ) ;
#193831=VECTOR ( 'NONE', #42923, 1000.000000000000000 ) ;
#194050=ADVANCED_FACE ( 'NONE', ( #30750 ), #60083, .T. ) ;
#194275=DIRECTION ( 'NONE',  ( 0.000000000000000000, 1.000000000000000000, 0.000000000000000000 ) ) ;
#194434=ORIENTED_EDGE ( 'NONE', *, *, #47118, .T. ) ;
#194512=DIRECTION ( 'NONE',  ( -1.000000000000000000, -0.000000000000000000, 0.000000000000000000 ) ) ;
#194517=ORIENTED_EDGE ( 'NONE', *, *, #157548, .T. ) ;
#194625=ORIENTED_EDGE ( 'NONE', *, *, #62627, .T. ) ;
#194990=DIRECTION ( 'NONE',  ( -0.000000000000000000, -0.6427876096865545730, -0.7660444431189654679 ) ) ;
#195579=CLOSED_SHELL ( 'NONE', ( #129135, #70778, #71148, #194050, #174806, #184460, #97292, #11482, #61485, #187386, #44161, #79380, #109611, #17861, #123330, #7466, #161836, #172508, #163302, #53964, #17963, #76561, #33975, #61711, #180856, #146491, #171353, #79813, #79289, #84282, #106136, #138616, #63761, #184302, #161701 ) ) ;
#195649=DIRECTION ( 'NONE',  ( 0.000000000000000000, -0.7660444431189836756, 0.6427876096865327016 ) ) ;
#195745=VECTOR ( 'NONE', #191448, 1000.000000000000000 ) ;
#195751=ORIENTED_EDGE ( 'NONE', *, *, #106434, .F. ) ;
#196475=ORIENTED_EDGE ( 'NONE', *, *, #58736, .F. ) ;
#196910=ORIENTED_EDGE ( 'NONE', *, *, #110318, .T. ) ;
#196981=VECTOR ( 'NONE', #31122, 1000.000000000000114 ) ;
#197216=VERTEX_POINT ( 'NONE', #109414 ) ;
#197470=LINE ( 'NONE', #14420, #56261 ) ;
#197703=DIRECTION ( 'NONE',  ( -1.000000000000000000, -0.000000000000000000, 0.000000000000000000 ) ) ;
#197771=ORIENTED_EDGE ( 'NONE', *, *, #92972, .F. ) ;
#198316=DIRECTION ( 'NONE',  ( 0.000000000000000000, 0.000000000000000000, 1.000000000000000000 ) ) ;
#198430=( GEOMETRIC_REPRESENTATION_CONTEXT ( 3 ) GLOBAL_UNCERTAINTY_ASSIGNED_CONTEXT ( ( #7444 ) ) GLOBAL_UNIT_ASSIGNED_CONTEXT ( ( #170444, #64259, #47107 ) ) REPRESENTATION_CONTEXT ( 'NONE', 'WORKASPACE' ) );
#198607=DIRECTION ( 'NONE',  ( -6.938893903907222067E-15, 0.000000000000000000, 1.000000000000000000 ) ) ;
#198827=EDGE_CURVE ( 'NONE', #1415, #143427, #75463, .T. ) ;
#198944=VERTEX_POINT ( 'NONE', #174836 ) ;
#199081=FACE_OUTER_BOUND ( 'NONE', #26835, .T. ) ;
#199247=PRESENTATION_STYLE_ASSIGNMENT (( #186075 ) ) ;
#199279=ORIENTED_EDGE ( 'NONE', *, *, #144774, .T. ) ;
#199314=DIRECTION ( 'NONE',  ( 0.000000000000000000, -1.000000000000000000, -0.000000000000000000 ) ) ;
#199327=DIRECTION ( 'NONE',  ( 1.000000000000000000, -0.000000000000000000, -0.000000000000000000 ) ) ;
#199430=DIRECTION ( 'NONE',  ( 0.000000000000000000, 0.000000000000000000, 1.000000000000000000 ) ) ;
#199571=DIRECTION ( 'NONE',  ( 0.000000000000000000, 1.000000000000000000, 0.000000000000000000 ) ) ;
#199587=ORIENTED_EDGE ( 'NONE', *, *, #8537, .F. ) ;
#199970=CARTESIAN_POINT ( 'NONE',  ( 4.500000000000000888, -140.0000000000000000, 22.27940468532398910 ) ) ;
ENDSEC;
END-ISO-10303-21;
